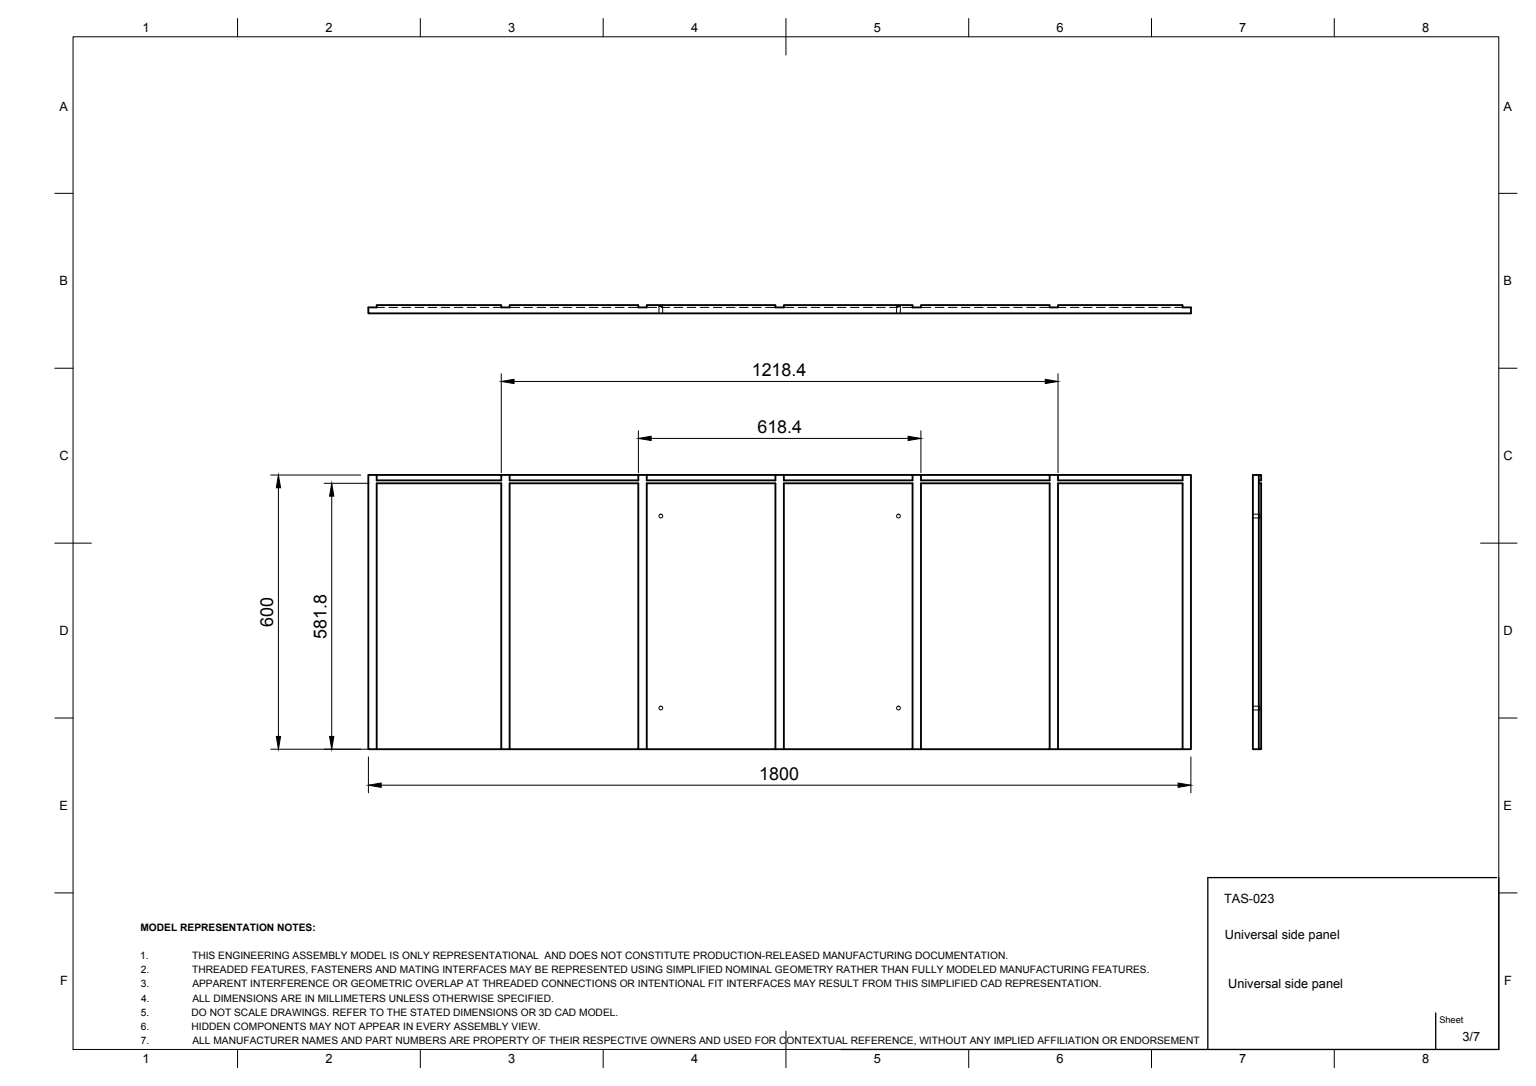
ISO-10303-21;
HEADER;
/* Generated by software containing ST-Developer
 * from STEP Tools, Inc. (www.steptools.com) 
 */

FILE_DESCRIPTION(
/* description */ (''),
/* implementation_level */ '2;1');

FILE_NAME(
/* name */ 'Universal side panel.step',
/* time_stamp */ '2026-11-15T17:51:54-08:00',
/* author */ (''),
/* organization */ (''),
/* preprocessor_version */ 'ST-DEVELOPER v20.2',
/* originating_system */ 'Autodesk Translation Framework v15.17.0.0',
/* authorisation */ '');

FILE_SCHEMA (('AUTOMOTIVE_DESIGN { 1 0 10303 214 3 1 1 }'));
ENDSEC;

DATA;
#10=MECHANICAL_DESIGN_GEOMETRIC_PRESENTATION_REPRESENTATION('',(#117),#2860);
#107=SHAPE_REPRESENTATION_RELATIONSHIP('SRR','None',#2902,#112);
#112=ADVANCED_BREP_SHAPE_REPRESENTATION('',(#122),#2855);
#117=STYLED_ITEM('',(#2936),#122);
#122=MANIFOLD_SOLID_BREP('Body1',#1714);
#127=FACE_BOUND('',#361,.T.);
#128=FACE_BOUND('',#362,.T.);
#129=FACE_BOUND('',#363,.T.);
#130=FACE_BOUND('',#364,.T.);
#131=PLANE('',#1780);
#132=PLANE('',#1784);
#133=PLANE('',#1788);
#134=PLANE('',#1792);
#135=PLANE('',#1793);
#136=PLANE('',#1794);
#137=PLANE('',#1795);
#138=PLANE('',#1796);
#139=PLANE('',#1797);
#140=PLANE('',#1798);
#141=PLANE('',#1799);
#142=PLANE('',#1800);
#143=PLANE('',#1801);
#144=PLANE('',#1802);
#145=PLANE('',#1803);
#146=PLANE('',#1804);
#147=PLANE('',#1805);
#148=PLANE('',#1806);
#149=PLANE('',#1807);
#150=PLANE('',#1808);
#151=PLANE('',#1809);
#152=PLANE('',#1810);
#153=PLANE('',#1811);
#154=PLANE('',#1812);
#155=PLANE('',#1813);
#156=PLANE('',#1814);
#157=PLANE('',#1815);
#158=PLANE('',#1816);
#159=PLANE('',#1817);
#160=PLANE('',#1818);
#161=PLANE('',#1819);
#162=PLANE('',#1820);
#163=PLANE('',#1821);
#164=PLANE('',#1822);
#165=PLANE('',#1823);
#166=PLANE('',#1824);
#167=PLANE('',#1825);
#168=PLANE('',#1826);
#169=PLANE('',#1827);
#170=PLANE('',#1828);
#171=PLANE('',#1829);
#172=PLANE('',#1830);
#173=PLANE('',#1831);
#174=PLANE('',#1832);
#175=PLANE('',#1833);
#176=PLANE('',#1834);
#177=PLANE('',#1835);
#178=PLANE('',#1836);
#179=PLANE('',#1837);
#180=PLANE('',#1838);
#181=PLANE('',#1839);
#182=PLANE('',#1840);
#183=PLANE('',#1841);
#184=PLANE('',#1842);
#185=PLANE('',#1843);
#186=PLANE('',#1844);
#187=PLANE('',#1845);
#188=PLANE('',#1846);
#213=FACE_OUTER_BOUND('',#300,.T.);
#214=FACE_OUTER_BOUND('',#301,.T.);
#215=FACE_OUTER_BOUND('',#302,.T.);
#216=FACE_OUTER_BOUND('',#303,.T.);
#217=FACE_OUTER_BOUND('',#304,.T.);
#218=FACE_OUTER_BOUND('',#305,.T.);
#219=FACE_OUTER_BOUND('',#306,.T.);
#220=FACE_OUTER_BOUND('',#307,.T.);
#221=FACE_OUTER_BOUND('',#308,.T.);
#222=FACE_OUTER_BOUND('',#309,.T.);
#223=FACE_OUTER_BOUND('',#310,.T.);
#224=FACE_OUTER_BOUND('',#311,.T.);
#225=FACE_OUTER_BOUND('',#312,.T.);
#226=FACE_OUTER_BOUND('',#313,.T.);
#227=FACE_OUTER_BOUND('',#314,.T.);
#228=FACE_OUTER_BOUND('',#315,.T.);
#229=FACE_OUTER_BOUND('',#316,.T.);
#230=FACE_OUTER_BOUND('',#317,.T.);
#231=FACE_OUTER_BOUND('',#318,.T.);
#232=FACE_OUTER_BOUND('',#319,.T.);
#233=FACE_OUTER_BOUND('',#320,.T.);
#234=FACE_OUTER_BOUND('',#321,.T.);
#235=FACE_OUTER_BOUND('',#322,.T.);
#236=FACE_OUTER_BOUND('',#323,.T.);
#237=FACE_OUTER_BOUND('',#324,.T.);
#238=FACE_OUTER_BOUND('',#325,.T.);
#239=FACE_OUTER_BOUND('',#326,.T.);
#240=FACE_OUTER_BOUND('',#327,.T.);
#241=FACE_OUTER_BOUND('',#328,.T.);
#242=FACE_OUTER_BOUND('',#329,.T.);
#243=FACE_OUTER_BOUND('',#330,.T.);
#244=FACE_OUTER_BOUND('',#331,.T.);
#245=FACE_OUTER_BOUND('',#332,.T.);
#246=FACE_OUTER_BOUND('',#333,.T.);
#247=FACE_OUTER_BOUND('',#334,.T.);
#248=FACE_OUTER_BOUND('',#335,.T.);
#249=FACE_OUTER_BOUND('',#336,.T.);
#250=FACE_OUTER_BOUND('',#337,.T.);
#251=FACE_OUTER_BOUND('',#338,.T.);
#252=FACE_OUTER_BOUND('',#339,.T.);
#253=FACE_OUTER_BOUND('',#340,.T.);
#254=FACE_OUTER_BOUND('',#341,.T.);
#255=FACE_OUTER_BOUND('',#342,.T.);
#256=FACE_OUTER_BOUND('',#343,.T.);
#257=FACE_OUTER_BOUND('',#344,.T.);
#258=FACE_OUTER_BOUND('',#345,.T.);
#259=FACE_OUTER_BOUND('',#346,.T.);
#260=FACE_OUTER_BOUND('',#347,.T.);
#261=FACE_OUTER_BOUND('',#348,.T.);
#262=FACE_OUTER_BOUND('',#349,.T.);
#263=FACE_OUTER_BOUND('',#350,.T.);
#264=FACE_OUTER_BOUND('',#351,.T.);
#265=FACE_OUTER_BOUND('',#352,.T.);
#266=FACE_OUTER_BOUND('',#353,.T.);
#267=FACE_OUTER_BOUND('',#354,.T.);
#268=FACE_OUTER_BOUND('',#355,.T.);
#269=FACE_OUTER_BOUND('',#356,.T.);
#270=FACE_OUTER_BOUND('',#357,.T.);
#271=FACE_OUTER_BOUND('',#358,.T.);
#272=FACE_OUTER_BOUND('',#359,.T.);
#273=FACE_OUTER_BOUND('',#360,.T.);
#274=FACE_OUTER_BOUND('',#365,.T.);
#300=EDGE_LOOP('',(#1184,#1185,#1186,#1187));
#301=EDGE_LOOP('',(#1188));
#302=EDGE_LOOP('',(#1189,#1190,#1191,#1192));
#303=EDGE_LOOP('',(#1193));
#304=EDGE_LOOP('',(#1194,#1195,#1196,#1197));
#305=EDGE_LOOP('',(#1198));
#306=EDGE_LOOP('',(#1199,#1200,#1201,#1202));
#307=EDGE_LOOP('',(#1203));
#308=EDGE_LOOP('',(#1204,#1205,#1206,#1207));
#309=EDGE_LOOP('',(#1208,#1209,#1210,#1211));
#310=EDGE_LOOP('',(#1212,#1213,#1214,#1215));
#311=EDGE_LOOP('',(#1216,#1217,#1218,#1219));
#312=EDGE_LOOP('',(#1220,#1221,#1222,#1223));
#313=EDGE_LOOP('',(#1224,#1225,#1226,#1227));
#314=EDGE_LOOP('',(#1228,#1229,#1230,#1231));
#315=EDGE_LOOP('',(#1232,#1233,#1234,#1235));
#316=EDGE_LOOP('',(#1236,#1237,#1238,#1239));
#317=EDGE_LOOP('',(#1240,#1241,#1242,#1243));
#318=EDGE_LOOP('',(#1244,#1245,#1246,#1247));
#319=EDGE_LOOP('',(#1248,#1249,#1250,#1251));
#320=EDGE_LOOP('',(#1252,#1253,#1254,#1255,#1256,#1257,#1258,#1259,#1260,
#1261,#1262,#1263,#1264,#1265,#1266,#1267,#1268,#1269,#1270,#1271,#1272,
#1273,#1274,#1275,#1276,#1277,#1278,#1279,#1280,#1281,#1282,#1283,#1284,
#1285,#1286,#1287,#1288,#1289,#1290,#1291,#1292,#1293,#1294,#1295,#1296,
#1297,#1298,#1299,#1300,#1301,#1302,#1303));
#321=EDGE_LOOP('',(#1304,#1305,#1306,#1307));
#322=EDGE_LOOP('',(#1308,#1309,#1310,#1311));
#323=EDGE_LOOP('',(#1312,#1313,#1314,#1315));
#324=EDGE_LOOP('',(#1316,#1317,#1318,#1319));
#325=EDGE_LOOP('',(#1320,#1321,#1322,#1323));
#326=EDGE_LOOP('',(#1324,#1325,#1326,#1327));
#327=EDGE_LOOP('',(#1328,#1329,#1330,#1331));
#328=EDGE_LOOP('',(#1332,#1333,#1334,#1335));
#329=EDGE_LOOP('',(#1336,#1337,#1338,#1339));
#330=EDGE_LOOP('',(#1340,#1341,#1342,#1343));
#331=EDGE_LOOP('',(#1344,#1345,#1346,#1347));
#332=EDGE_LOOP('',(#1348,#1349,#1350,#1351));
#333=EDGE_LOOP('',(#1352,#1353,#1354,#1355));
#334=EDGE_LOOP('',(#1356,#1357,#1358,#1359));
#335=EDGE_LOOP('',(#1360,#1361,#1362,#1363));
#336=EDGE_LOOP('',(#1364,#1365,#1366,#1367));
#337=EDGE_LOOP('',(#1368,#1369,#1370,#1371));
#338=EDGE_LOOP('',(#1372,#1373,#1374,#1375));
#339=EDGE_LOOP('',(#1376,#1377,#1378,#1379));
#340=EDGE_LOOP('',(#1380,#1381,#1382,#1383));
#341=EDGE_LOOP('',(#1384,#1385,#1386,#1387));
#342=EDGE_LOOP('',(#1388,#1389,#1390,#1391));
#343=EDGE_LOOP('',(#1392,#1393,#1394,#1395));
#344=EDGE_LOOP('',(#1396,#1397,#1398,#1399));
#345=EDGE_LOOP('',(#1400,#1401,#1402,#1403));
#346=EDGE_LOOP('',(#1404,#1405,#1406,#1407));
#347=EDGE_LOOP('',(#1408,#1409,#1410,#1411));
#348=EDGE_LOOP('',(#1412,#1413,#1414,#1415));
#349=EDGE_LOOP('',(#1416,#1417,#1418,#1419));
#350=EDGE_LOOP('',(#1420,#1421,#1422,#1423));
#351=EDGE_LOOP('',(#1424,#1425,#1426,#1427));
#352=EDGE_LOOP('',(#1428,#1429,#1430,#1431));
#353=EDGE_LOOP('',(#1432,#1433,#1434,#1435));
#354=EDGE_LOOP('',(#1436,#1437,#1438,#1439));
#355=EDGE_LOOP('',(#1440,#1441,#1442,#1443));
#356=EDGE_LOOP('',(#1444,#1445,#1446,#1447));
#357=EDGE_LOOP('',(#1448,#1449,#1450,#1451,#1452,#1453,#1454,#1455,#1456,
#1457,#1458,#1459,#1460,#1461,#1462,#1463,#1464,#1465,#1466,#1467,#1468,
#1469,#1470,#1471,#1472,#1473,#1474,#1475));
#358=EDGE_LOOP('',(#1476,#1477,#1478,#1479));
#359=EDGE_LOOP('',(#1480,#1481,#1482,#1483,#1484,#1485,#1486,#1487,#1488,
#1489,#1490,#1491,#1492,#1493,#1494,#1495,#1496,#1497,#1498,#1499,#1500,
#1501,#1502,#1503,#1504,#1505,#1506,#1507));
#360=EDGE_LOOP('',(#1508,#1509,#1510,#1511));
#361=EDGE_LOOP('',(#1512));
#362=EDGE_LOOP('',(#1513));
#363=EDGE_LOOP('',(#1514));
#364=EDGE_LOOP('',(#1515));
#365=EDGE_LOOP('',(#1516,#1517,#1518,#1519));
#391=LINE('',#2371,#600);
#392=LINE('',#2378,#601);
#393=LINE('',#2385,#602);
#394=LINE('',#2392,#603);
#395=LINE('',#2398,#604);
#396=LINE('',#2400,#605);
#397=LINE('',#2402,#606);
#398=LINE('',#2403,#607);
#399=LINE('',#2407,#608);
#400=LINE('',#2409,#609);
#401=LINE('',#2411,#610);
#402=LINE('',#2412,#611);
#403=LINE('',#2416,#612);
#404=LINE('',#2418,#613);
#405=LINE('',#2420,#614);
#406=LINE('',#2421,#615);
#407=LINE('',#2425,#616);
#408=LINE('',#2427,#617);
#409=LINE('',#2429,#618);
#410=LINE('',#2430,#619);
#411=LINE('',#2434,#620);
#412=LINE('',#2436,#621);
#413=LINE('',#2438,#622);
#414=LINE('',#2439,#623);
#415=LINE('',#2443,#624);
#416=LINE('',#2445,#625);
#417=LINE('',#2447,#626);
#418=LINE('',#2448,#627);
#419=LINE('',#2452,#628);
#420=LINE('',#2454,#629);
#421=LINE('',#2456,#630);
#422=LINE('',#2457,#631);
#423=LINE('',#2461,#632);
#424=LINE('',#2463,#633);
#425=LINE('',#2465,#634);
#426=LINE('',#2466,#635);
#427=LINE('',#2470,#636);
#428=LINE('',#2472,#637);
#429=LINE('',#2474,#638);
#430=LINE('',#2475,#639);
#431=LINE('',#2479,#640);
#432=LINE('',#2481,#641);
#433=LINE('',#2483,#642);
#434=LINE('',#2484,#643);
#435=LINE('',#2488,#644);
#436=LINE('',#2490,#645);
#437=LINE('',#2492,#646);
#438=LINE('',#2493,#647);
#439=LINE('',#2497,#648);
#440=LINE('',#2499,#649);
#441=LINE('',#2501,#650);
#442=LINE('',#2502,#651);
#443=LINE('',#2505,#652);
#444=LINE('',#2507,#653);
#445=LINE('',#2509,#654);
#446=LINE('',#2511,#655);
#447=LINE('',#2512,#656);
#448=LINE('',#2514,#657);
#449=LINE('',#2516,#658);
#450=LINE('',#2517,#659);
#451=LINE('',#2519,#660);
#452=LINE('',#2521,#661);
#453=LINE('',#2522,#662);
#454=LINE('',#2524,#663);
#455=LINE('',#2526,#664);
#456=LINE('',#2527,#665);
#457=LINE('',#2529,#666);
#458=LINE('',#2531,#667);
#459=LINE('',#2532,#668);
#460=LINE('',#2534,#669);
#461=LINE('',#2536,#670);
#462=LINE('',#2537,#671);
#463=LINE('',#2539,#672);
#464=LINE('',#2541,#673);
#465=LINE('',#2543,#674);
#466=LINE('',#2545,#675);
#467=LINE('',#2546,#676);
#468=LINE('',#2548,#677);
#469=LINE('',#2550,#678);
#470=LINE('',#2551,#679);
#471=LINE('',#2553,#680);
#472=LINE('',#2555,#681);
#473=LINE('',#2556,#682);
#474=LINE('',#2558,#683);
#475=LINE('',#2560,#684);
#476=LINE('',#2561,#685);
#477=LINE('',#2563,#686);
#478=LINE('',#2565,#687);
#479=LINE('',#2566,#688);
#480=LINE('',#2568,#689);
#481=LINE('',#2570,#690);
#482=LINE('',#2571,#691);
#483=LINE('',#2574,#692);
#484=LINE('',#2575,#693);
#485=LINE('',#2578,#694);
#486=LINE('',#2579,#695);
#487=LINE('',#2582,#696);
#488=LINE('',#2583,#697);
#489=LINE('',#2586,#698);
#490=LINE('',#2587,#699);
#491=LINE('',#2589,#700);
#492=LINE('',#2591,#701);
#493=LINE('',#2594,#702);
#494=LINE('',#2595,#703);
#495=LINE('',#2598,#704);
#496=LINE('',#2599,#705);
#497=LINE('',#2602,#706);
#498=LINE('',#2603,#707);
#499=LINE('',#2606,#708);
#500=LINE('',#2607,#709);
#501=LINE('',#2609,#710);
#502=LINE('',#2611,#711);
#503=LINE('',#2614,#712);
#504=LINE('',#2615,#713);
#505=LINE('',#2618,#714);
#506=LINE('',#2619,#715);
#507=LINE('',#2622,#716);
#508=LINE('',#2623,#717);
#509=LINE('',#2626,#718);
#510=LINE('',#2627,#719);
#511=LINE('',#2629,#720);
#512=LINE('',#2631,#721);
#513=LINE('',#2634,#722);
#514=LINE('',#2635,#723);
#515=LINE('',#2638,#724);
#516=LINE('',#2639,#725);
#517=LINE('',#2642,#726);
#518=LINE('',#2643,#727);
#519=LINE('',#2646,#728);
#520=LINE('',#2647,#729);
#521=LINE('',#2649,#730);
#522=LINE('',#2651,#731);
#523=LINE('',#2654,#732);
#524=LINE('',#2655,#733);
#525=LINE('',#2658,#734);
#526=LINE('',#2659,#735);
#527=LINE('',#2662,#736);
#528=LINE('',#2663,#737);
#529=LINE('',#2666,#738);
#530=LINE('',#2667,#739);
#531=LINE('',#2669,#740);
#532=LINE('',#2671,#741);
#533=LINE('',#2674,#742);
#534=LINE('',#2675,#743);
#535=LINE('',#2678,#744);
#536=LINE('',#2679,#745);
#537=LINE('',#2682,#746);
#538=LINE('',#2683,#747);
#539=LINE('',#2686,#748);
#540=LINE('',#2687,#749);
#541=LINE('',#2689,#750);
#542=LINE('',#2691,#751);
#543=LINE('',#2694,#752);
#544=LINE('',#2696,#753);
#545=LINE('',#2697,#754);
#546=LINE('',#2700,#755);
#547=LINE('',#2701,#756);
#548=LINE('',#2704,#757);
#549=LINE('',#2705,#758);
#550=LINE('',#2707,#759);
#600=VECTOR('',#1910,0.409999999999997);
#601=VECTOR('',#1919,0.409999999999997);
#602=VECTOR('',#1928,0.409999999999997);
#603=VECTOR('',#1937,0.409999999999997);
#604=VECTOR('',#1944,1.);
#605=VECTOR('',#1945,1.);
#606=VECTOR('',#1946,1.);
#607=VECTOR('',#1947,1.);
#608=VECTOR('',#1950,1.);
#609=VECTOR('',#1951,1.);
#610=VECTOR('',#1952,1.);
#611=VECTOR('',#1953,1.);
#612=VECTOR('',#1956,1.);
#613=VECTOR('',#1957,1.);
#614=VECTOR('',#1958,1.);
#615=VECTOR('',#1959,1.);
#616=VECTOR('',#1962,1.);
#617=VECTOR('',#1963,1.);
#618=VECTOR('',#1964,1.);
#619=VECTOR('',#1965,1.);
#620=VECTOR('',#1968,1.);
#621=VECTOR('',#1969,1.);
#622=VECTOR('',#1970,1.);
#623=VECTOR('',#1971,1.);
#624=VECTOR('',#1974,1.);
#625=VECTOR('',#1975,1.);
#626=VECTOR('',#1976,1.);
#627=VECTOR('',#1977,1.);
#628=VECTOR('',#1980,1.);
#629=VECTOR('',#1981,1.);
#630=VECTOR('',#1982,1.);
#631=VECTOR('',#1983,1.);
#632=VECTOR('',#1986,1.);
#633=VECTOR('',#1987,1.);
#634=VECTOR('',#1988,1.);
#635=VECTOR('',#1989,1.);
#636=VECTOR('',#1992,1.);
#637=VECTOR('',#1993,1.);
#638=VECTOR('',#1994,1.);
#639=VECTOR('',#1995,1.);
#640=VECTOR('',#1998,1.);
#641=VECTOR('',#1999,1.);
#642=VECTOR('',#2000,1.);
#643=VECTOR('',#2001,1.);
#644=VECTOR('',#2004,1.);
#645=VECTOR('',#2005,1.);
#646=VECTOR('',#2006,1.);
#647=VECTOR('',#2007,1.);
#648=VECTOR('',#2010,1.);
#649=VECTOR('',#2011,1.);
#650=VECTOR('',#2012,1.);
#651=VECTOR('',#2013,1.);
#652=VECTOR('',#2016,1.);
#653=VECTOR('',#2017,1.);
#654=VECTOR('',#2018,1.);
#655=VECTOR('',#2019,1.);
#656=VECTOR('',#2020,1.);
#657=VECTOR('',#2021,1.);
#658=VECTOR('',#2022,1.);
#659=VECTOR('',#2023,1.);
#660=VECTOR('',#2024,1.);
#661=VECTOR('',#2025,1.);
#662=VECTOR('',#2026,1.);
#663=VECTOR('',#2027,1.);
#664=VECTOR('',#2028,1.);
#665=VECTOR('',#2029,1.);
#666=VECTOR('',#2030,1.);
#667=VECTOR('',#2031,1.);
#668=VECTOR('',#2032,1.);
#669=VECTOR('',#2033,1.);
#670=VECTOR('',#2034,1.);
#671=VECTOR('',#2035,1.);
#672=VECTOR('',#2036,1.);
#673=VECTOR('',#2037,1.);
#674=VECTOR('',#2038,1.);
#675=VECTOR('',#2039,1.);
#676=VECTOR('',#2040,1.);
#677=VECTOR('',#2041,1.);
#678=VECTOR('',#2042,1.);
#679=VECTOR('',#2043,1.);
#680=VECTOR('',#2044,1.);
#681=VECTOR('',#2045,1.);
#682=VECTOR('',#2046,1.);
#683=VECTOR('',#2047,1.);
#684=VECTOR('',#2048,1.);
#685=VECTOR('',#2049,1.);
#686=VECTOR('',#2050,1.);
#687=VECTOR('',#2051,1.);
#688=VECTOR('',#2052,1.);
#689=VECTOR('',#2053,1.);
#690=VECTOR('',#2054,1.);
#691=VECTOR('',#2055,1.);
#692=VECTOR('',#2058,1.);
#693=VECTOR('',#2059,1.);
#694=VECTOR('',#2062,1.);
#695=VECTOR('',#2063,1.);
#696=VECTOR('',#2066,1.);
#697=VECTOR('',#2067,1.);
#698=VECTOR('',#2070,1.);
#699=VECTOR('',#2071,1.);
#700=VECTOR('',#2074,1.);
#701=VECTOR('',#2077,1.);
#702=VECTOR('',#2080,1.);
#703=VECTOR('',#2081,1.);
#704=VECTOR('',#2084,1.);
#705=VECTOR('',#2085,1.);
#706=VECTOR('',#2088,1.);
#707=VECTOR('',#2089,1.);
#708=VECTOR('',#2092,1.);
#709=VECTOR('',#2093,1.);
#710=VECTOR('',#2096,1.);
#711=VECTOR('',#2099,1.);
#712=VECTOR('',#2102,1.);
#713=VECTOR('',#2103,1.);
#714=VECTOR('',#2106,1.);
#715=VECTOR('',#2107,1.);
#716=VECTOR('',#2110,1.);
#717=VECTOR('',#2111,1.);
#718=VECTOR('',#2114,1.);
#719=VECTOR('',#2115,1.);
#720=VECTOR('',#2118,1.);
#721=VECTOR('',#2121,1.);
#722=VECTOR('',#2124,1.);
#723=VECTOR('',#2125,1.);
#724=VECTOR('',#2128,1.);
#725=VECTOR('',#2129,1.);
#726=VECTOR('',#2132,1.);
#727=VECTOR('',#2133,1.);
#728=VECTOR('',#2136,1.);
#729=VECTOR('',#2137,1.);
#730=VECTOR('',#2140,1.);
#731=VECTOR('',#2143,1.);
#732=VECTOR('',#2146,1.);
#733=VECTOR('',#2147,1.);
#734=VECTOR('',#2150,1.);
#735=VECTOR('',#2151,1.);
#736=VECTOR('',#2154,1.);
#737=VECTOR('',#2155,1.);
#738=VECTOR('',#2158,1.);
#739=VECTOR('',#2159,1.);
#740=VECTOR('',#2162,1.);
#741=VECTOR('',#2165,1.);
#742=VECTOR('',#2168,1.);
#743=VECTOR('',#2169,1.);
#744=VECTOR('',#2172,1.);
#745=VECTOR('',#2173,1.);
#746=VECTOR('',#2176,1.);
#747=VECTOR('',#2177,1.);
#748=VECTOR('',#2180,1.);
#749=VECTOR('',#2181,1.);
#750=VECTOR('',#2184,1.);
#751=VECTOR('',#2187,1.);
#752=VECTOR('',#2190,1.);
#753=VECTOR('',#2191,1.);
#754=VECTOR('',#2192,1.);
#755=VECTOR('',#2195,1.);
#756=VECTOR('',#2196,1.);
#757=VECTOR('',#2199,1.);
#758=VECTOR('',#2200,1.);
#759=VECTOR('',#2203,1.);
#809=CIRCLE('',#1778,0.409999999999997);
#810=CIRCLE('',#1779,0.409999999999997);
#811=CIRCLE('',#1782,0.409999999999997);
#812=CIRCLE('',#1783,0.409999999999997);
#813=CIRCLE('',#1786,0.409999999999997);
#814=CIRCLE('',#1787,0.409999999999997);
#815=CIRCLE('',#1790,0.409999999999997);
#816=CIRCLE('',#1791,0.409999999999997);
#819=VERTEX_POINT('',#2368);
#820=VERTEX_POINT('',#2370);
#821=VERTEX_POINT('',#2375);
#822=VERTEX_POINT('',#2377);
#823=VERTEX_POINT('',#2382);
#824=VERTEX_POINT('',#2384);
#825=VERTEX_POINT('',#2389);
#826=VERTEX_POINT('',#2391);
#827=VERTEX_POINT('',#2396);
#828=VERTEX_POINT('',#2397);
#829=VERTEX_POINT('',#2399);
#830=VERTEX_POINT('',#2401);
#831=VERTEX_POINT('',#2405);
#832=VERTEX_POINT('',#2406);
#833=VERTEX_POINT('',#2408);
#834=VERTEX_POINT('',#2410);
#835=VERTEX_POINT('',#2414);
#836=VERTEX_POINT('',#2415);
#837=VERTEX_POINT('',#2417);
#838=VERTEX_POINT('',#2419);
#839=VERTEX_POINT('',#2423);
#840=VERTEX_POINT('',#2424);
#841=VERTEX_POINT('',#2426);
#842=VERTEX_POINT('',#2428);
#843=VERTEX_POINT('',#2432);
#844=VERTEX_POINT('',#2433);
#845=VERTEX_POINT('',#2435);
#846=VERTEX_POINT('',#2437);
#847=VERTEX_POINT('',#2441);
#848=VERTEX_POINT('',#2442);
#849=VERTEX_POINT('',#2444);
#850=VERTEX_POINT('',#2446);
#851=VERTEX_POINT('',#2450);
#852=VERTEX_POINT('',#2451);
#853=VERTEX_POINT('',#2453);
#854=VERTEX_POINT('',#2455);
#855=VERTEX_POINT('',#2459);
#856=VERTEX_POINT('',#2460);
#857=VERTEX_POINT('',#2462);
#858=VERTEX_POINT('',#2464);
#859=VERTEX_POINT('',#2468);
#860=VERTEX_POINT('',#2469);
#861=VERTEX_POINT('',#2471);
#862=VERTEX_POINT('',#2473);
#863=VERTEX_POINT('',#2477);
#864=VERTEX_POINT('',#2478);
#865=VERTEX_POINT('',#2480);
#866=VERTEX_POINT('',#2482);
#867=VERTEX_POINT('',#2486);
#868=VERTEX_POINT('',#2487);
#869=VERTEX_POINT('',#2489);
#870=VERTEX_POINT('',#2491);
#871=VERTEX_POINT('',#2495);
#872=VERTEX_POINT('',#2496);
#873=VERTEX_POINT('',#2498);
#874=VERTEX_POINT('',#2500);
#875=VERTEX_POINT('',#2504);
#876=VERTEX_POINT('',#2506);
#877=VERTEX_POINT('',#2508);
#878=VERTEX_POINT('',#2510);
#879=VERTEX_POINT('',#2513);
#880=VERTEX_POINT('',#2515);
#881=VERTEX_POINT('',#2518);
#882=VERTEX_POINT('',#2520);
#883=VERTEX_POINT('',#2523);
#884=VERTEX_POINT('',#2525);
#885=VERTEX_POINT('',#2528);
#886=VERTEX_POINT('',#2530);
#887=VERTEX_POINT('',#2533);
#888=VERTEX_POINT('',#2535);
#889=VERTEX_POINT('',#2538);
#890=VERTEX_POINT('',#2540);
#891=VERTEX_POINT('',#2542);
#892=VERTEX_POINT('',#2544);
#893=VERTEX_POINT('',#2547);
#894=VERTEX_POINT('',#2549);
#895=VERTEX_POINT('',#2552);
#896=VERTEX_POINT('',#2554);
#897=VERTEX_POINT('',#2557);
#898=VERTEX_POINT('',#2559);
#899=VERTEX_POINT('',#2562);
#900=VERTEX_POINT('',#2564);
#901=VERTEX_POINT('',#2567);
#902=VERTEX_POINT('',#2569);
#903=VERTEX_POINT('',#2573);
#904=VERTEX_POINT('',#2577);
#905=VERTEX_POINT('',#2581);
#906=VERTEX_POINT('',#2585);
#907=VERTEX_POINT('',#2593);
#908=VERTEX_POINT('',#2597);
#909=VERTEX_POINT('',#2601);
#910=VERTEX_POINT('',#2605);
#911=VERTEX_POINT('',#2613);
#912=VERTEX_POINT('',#2617);
#913=VERTEX_POINT('',#2621);
#914=VERTEX_POINT('',#2625);
#915=VERTEX_POINT('',#2633);
#916=VERTEX_POINT('',#2637);
#917=VERTEX_POINT('',#2641);
#918=VERTEX_POINT('',#2645);
#919=VERTEX_POINT('',#2653);
#920=VERTEX_POINT('',#2657);
#921=VERTEX_POINT('',#2661);
#922=VERTEX_POINT('',#2665);
#923=VERTEX_POINT('',#2673);
#924=VERTEX_POINT('',#2677);
#925=VERTEX_POINT('',#2681);
#926=VERTEX_POINT('',#2685);
#927=VERTEX_POINT('',#2693);
#928=VERTEX_POINT('',#2695);
#929=VERTEX_POINT('',#2699);
#930=VERTEX_POINT('',#2703);
#965=EDGE_CURVE('',#819,#819,#809,.T.);
#966=EDGE_CURVE('',#819,#820,#391,.T.);
#967=EDGE_CURVE('',#820,#820,#810,.T.);
#968=EDGE_CURVE('',#821,#821,#811,.T.);
#969=EDGE_CURVE('',#821,#822,#392,.T.);
#970=EDGE_CURVE('',#822,#822,#812,.T.);
#971=EDGE_CURVE('',#823,#823,#813,.T.);
#972=EDGE_CURVE('',#823,#824,#393,.T.);
#973=EDGE_CURVE('',#824,#824,#814,.T.);
#974=EDGE_CURVE('',#825,#825,#815,.T.);
#975=EDGE_CURVE('',#825,#826,#394,.T.);
#976=EDGE_CURVE('',#826,#826,#816,.T.);
#977=EDGE_CURVE('',#827,#828,#395,.T.);
#978=EDGE_CURVE('',#829,#827,#396,.T.);
#979=EDGE_CURVE('',#830,#829,#397,.T.);
#980=EDGE_CURVE('',#828,#830,#398,.T.);
#981=EDGE_CURVE('',#831,#832,#399,.T.);
#982=EDGE_CURVE('',#833,#831,#400,.T.);
#983=EDGE_CURVE('',#834,#833,#401,.T.);
#984=EDGE_CURVE('',#832,#834,#402,.T.);
#985=EDGE_CURVE('',#835,#836,#403,.T.);
#986=EDGE_CURVE('',#837,#835,#404,.T.);
#987=EDGE_CURVE('',#838,#837,#405,.T.);
#988=EDGE_CURVE('',#836,#838,#406,.T.);
#989=EDGE_CURVE('',#839,#840,#407,.T.);
#990=EDGE_CURVE('',#841,#839,#408,.T.);
#991=EDGE_CURVE('',#842,#841,#409,.T.);
#992=EDGE_CURVE('',#840,#842,#410,.T.);
#993=EDGE_CURVE('',#843,#844,#411,.T.);
#994=EDGE_CURVE('',#845,#843,#412,.T.);
#995=EDGE_CURVE('',#846,#845,#413,.T.);
#996=EDGE_CURVE('',#844,#846,#414,.T.);
#997=EDGE_CURVE('',#847,#848,#415,.T.);
#998=EDGE_CURVE('',#849,#847,#416,.T.);
#999=EDGE_CURVE('',#850,#849,#417,.T.);
#1000=EDGE_CURVE('',#848,#850,#418,.T.);
#1001=EDGE_CURVE('',#851,#852,#419,.T.);
#1002=EDGE_CURVE('',#853,#851,#420,.T.);
#1003=EDGE_CURVE('',#854,#853,#421,.T.);
#1004=EDGE_CURVE('',#854,#852,#422,.T.);
#1005=EDGE_CURVE('',#855,#856,#423,.T.);
#1006=EDGE_CURVE('',#857,#855,#424,.T.);
#1007=EDGE_CURVE('',#858,#857,#425,.T.);
#1008=EDGE_CURVE('',#858,#856,#426,.T.);
#1009=EDGE_CURVE('',#859,#860,#427,.T.);
#1010=EDGE_CURVE('',#861,#859,#428,.T.);
#1011=EDGE_CURVE('',#862,#861,#429,.T.);
#1012=EDGE_CURVE('',#862,#860,#430,.T.);
#1013=EDGE_CURVE('',#863,#864,#431,.T.);
#1014=EDGE_CURVE('',#865,#863,#432,.T.);
#1015=EDGE_CURVE('',#866,#865,#433,.T.);
#1016=EDGE_CURVE('',#866,#864,#434,.T.);
#1017=EDGE_CURVE('',#867,#868,#435,.T.);
#1018=EDGE_CURVE('',#869,#867,#436,.T.);
#1019=EDGE_CURVE('',#870,#869,#437,.T.);
#1020=EDGE_CURVE('',#870,#868,#438,.T.);
#1021=EDGE_CURVE('',#871,#872,#439,.T.);
#1022=EDGE_CURVE('',#873,#871,#440,.T.);
#1023=EDGE_CURVE('',#874,#873,#441,.T.);
#1024=EDGE_CURVE('',#874,#872,#442,.T.);
#1025=EDGE_CURVE('',#875,#847,#443,.T.);
#1026=EDGE_CURVE('',#876,#875,#444,.T.);
#1027=EDGE_CURVE('',#877,#876,#445,.T.);
#1028=EDGE_CURVE('',#878,#877,#446,.T.);
#1029=EDGE_CURVE('',#872,#878,#447,.T.);
#1030=EDGE_CURVE('',#874,#879,#448,.T.);
#1031=EDGE_CURVE('',#880,#879,#449,.T.);
#1032=EDGE_CURVE('',#868,#880,#450,.T.);
#1033=EDGE_CURVE('',#870,#881,#451,.T.);
#1034=EDGE_CURVE('',#882,#881,#452,.T.);
#1035=EDGE_CURVE('',#864,#882,#453,.T.);
#1036=EDGE_CURVE('',#866,#883,#454,.T.);
#1037=EDGE_CURVE('',#884,#883,#455,.T.);
#1038=EDGE_CURVE('',#860,#884,#456,.T.);
#1039=EDGE_CURVE('',#862,#885,#457,.T.);
#1040=EDGE_CURVE('',#886,#885,#458,.T.);
#1041=EDGE_CURVE('',#856,#886,#459,.T.);
#1042=EDGE_CURVE('',#858,#887,#460,.T.);
#1043=EDGE_CURVE('',#888,#887,#461,.T.);
#1044=EDGE_CURVE('',#852,#888,#462,.T.);
#1045=EDGE_CURVE('',#854,#889,#463,.T.);
#1046=EDGE_CURVE('',#890,#889,#464,.T.);
#1047=EDGE_CURVE('',#891,#890,#465,.T.);
#1048=EDGE_CURVE('',#892,#891,#466,.T.);
#1049=EDGE_CURVE('',#892,#845,#467,.T.);
#1050=EDGE_CURVE('',#893,#843,#468,.T.);
#1051=EDGE_CURVE('',#894,#893,#469,.T.);
#1052=EDGE_CURVE('',#894,#841,#470,.T.);
#1053=EDGE_CURVE('',#895,#839,#471,.T.);
#1054=EDGE_CURVE('',#896,#895,#472,.T.);
#1055=EDGE_CURVE('',#896,#837,#473,.T.);
#1056=EDGE_CURVE('',#897,#835,#474,.T.);
#1057=EDGE_CURVE('',#898,#897,#475,.T.);
#1058=EDGE_CURVE('',#898,#833,#476,.T.);
#1059=EDGE_CURVE('',#899,#831,#477,.T.);
#1060=EDGE_CURVE('',#900,#899,#478,.T.);
#1061=EDGE_CURVE('',#900,#829,#479,.T.);
#1062=EDGE_CURVE('',#901,#827,#480,.T.);
#1063=EDGE_CURVE('',#902,#901,#481,.T.);
#1064=EDGE_CURVE('',#902,#849,#482,.T.);
#1065=EDGE_CURVE('',#903,#878,#483,.T.);
#1066=EDGE_CURVE('',#871,#903,#484,.T.);
#1067=EDGE_CURVE('',#904,#848,#485,.T.);
#1068=EDGE_CURVE('',#875,#904,#486,.T.);
#1069=EDGE_CURVE('',#905,#903,#487,.T.);
#1070=EDGE_CURVE('',#905,#873,#488,.T.);
#1071=EDGE_CURVE('',#850,#906,#489,.T.);
#1072=EDGE_CURVE('',#906,#904,#490,.T.);
#1073=EDGE_CURVE('',#879,#905,#491,.T.);
#1074=EDGE_CURVE('',#906,#902,#492,.T.);
#1075=EDGE_CURVE('',#907,#880,#493,.T.);
#1076=EDGE_CURVE('',#867,#907,#494,.T.);
#1077=EDGE_CURVE('',#908,#828,#495,.T.);
#1078=EDGE_CURVE('',#901,#908,#496,.T.);
#1079=EDGE_CURVE('',#909,#907,#497,.T.);
#1080=EDGE_CURVE('',#909,#869,#498,.T.);
#1081=EDGE_CURVE('',#830,#910,#499,.T.);
#1082=EDGE_CURVE('',#910,#908,#500,.T.);
#1083=EDGE_CURVE('',#881,#909,#501,.T.);
#1084=EDGE_CURVE('',#910,#900,#502,.T.);
#1085=EDGE_CURVE('',#911,#882,#503,.T.);
#1086=EDGE_CURVE('',#863,#911,#504,.T.);
#1087=EDGE_CURVE('',#912,#832,#505,.T.);
#1088=EDGE_CURVE('',#899,#912,#506,.T.);
#1089=EDGE_CURVE('',#913,#911,#507,.T.);
#1090=EDGE_CURVE('',#913,#865,#508,.T.);
#1091=EDGE_CURVE('',#834,#914,#509,.T.);
#1092=EDGE_CURVE('',#914,#912,#510,.T.);
#1093=EDGE_CURVE('',#883,#913,#511,.T.);
#1094=EDGE_CURVE('',#914,#898,#512,.T.);
#1095=EDGE_CURVE('',#915,#884,#513,.T.);
#1096=EDGE_CURVE('',#859,#915,#514,.T.);
#1097=EDGE_CURVE('',#916,#836,#515,.T.);
#1098=EDGE_CURVE('',#897,#916,#516,.T.);
#1099=EDGE_CURVE('',#917,#915,#517,.T.);
#1100=EDGE_CURVE('',#917,#861,#518,.T.);
#1101=EDGE_CURVE('',#838,#918,#519,.T.);
#1102=EDGE_CURVE('',#918,#916,#520,.T.);
#1103=EDGE_CURVE('',#885,#917,#521,.T.);
#1104=EDGE_CURVE('',#918,#896,#522,.T.);
#1105=EDGE_CURVE('',#919,#886,#523,.T.);
#1106=EDGE_CURVE('',#855,#919,#524,.T.);
#1107=EDGE_CURVE('',#920,#840,#525,.T.);
#1108=EDGE_CURVE('',#895,#920,#526,.T.);
#1109=EDGE_CURVE('',#921,#919,#527,.T.);
#1110=EDGE_CURVE('',#921,#857,#528,.T.);
#1111=EDGE_CURVE('',#842,#922,#529,.T.);
#1112=EDGE_CURVE('',#922,#920,#530,.T.);
#1113=EDGE_CURVE('',#887,#921,#531,.T.);
#1114=EDGE_CURVE('',#922,#894,#532,.T.);
#1115=EDGE_CURVE('',#923,#888,#533,.T.);
#1116=EDGE_CURVE('',#851,#923,#534,.T.);
#1117=EDGE_CURVE('',#924,#844,#535,.T.);
#1118=EDGE_CURVE('',#893,#924,#536,.T.);
#1119=EDGE_CURVE('',#925,#923,#537,.T.);
#1120=EDGE_CURVE('',#925,#853,#538,.T.);
#1121=EDGE_CURVE('',#846,#926,#539,.T.);
#1122=EDGE_CURVE('',#926,#924,#540,.T.);
#1123=EDGE_CURVE('',#889,#925,#541,.T.);
#1124=EDGE_CURVE('',#926,#892,#542,.T.);
#1125=EDGE_CURVE('',#891,#927,#543,.T.);
#1126=EDGE_CURVE('',#927,#928,#544,.T.);
#1127=EDGE_CURVE('',#876,#928,#545,.T.);
#1128=EDGE_CURVE('',#929,#890,#546,.T.);
#1129=EDGE_CURVE('',#927,#929,#547,.T.);
#1130=EDGE_CURVE('',#930,#877,#548,.T.);
#1131=EDGE_CURVE('',#929,#930,#549,.T.);
#1132=EDGE_CURVE('',#928,#930,#550,.T.);
#1184=ORIENTED_EDGE('',*,*,#965,.F.);
#1185=ORIENTED_EDGE('',*,*,#966,.T.);
#1186=ORIENTED_EDGE('',*,*,#967,.T.);
#1187=ORIENTED_EDGE('',*,*,#966,.F.);
#1188=ORIENTED_EDGE('',*,*,#967,.F.);
#1189=ORIENTED_EDGE('',*,*,#968,.F.);
#1190=ORIENTED_EDGE('',*,*,#969,.T.);
#1191=ORIENTED_EDGE('',*,*,#970,.T.);
#1192=ORIENTED_EDGE('',*,*,#969,.F.);
#1193=ORIENTED_EDGE('',*,*,#970,.F.);
#1194=ORIENTED_EDGE('',*,*,#971,.F.);
#1195=ORIENTED_EDGE('',*,*,#972,.T.);
#1196=ORIENTED_EDGE('',*,*,#973,.T.);
#1197=ORIENTED_EDGE('',*,*,#972,.F.);
#1198=ORIENTED_EDGE('',*,*,#973,.F.);
#1199=ORIENTED_EDGE('',*,*,#974,.F.);
#1200=ORIENTED_EDGE('',*,*,#975,.T.);
#1201=ORIENTED_EDGE('',*,*,#976,.T.);
#1202=ORIENTED_EDGE('',*,*,#975,.F.);
#1203=ORIENTED_EDGE('',*,*,#976,.F.);
#1204=ORIENTED_EDGE('',*,*,#977,.F.);
#1205=ORIENTED_EDGE('',*,*,#978,.F.);
#1206=ORIENTED_EDGE('',*,*,#979,.F.);
#1207=ORIENTED_EDGE('',*,*,#980,.F.);
#1208=ORIENTED_EDGE('',*,*,#981,.F.);
#1209=ORIENTED_EDGE('',*,*,#982,.F.);
#1210=ORIENTED_EDGE('',*,*,#983,.F.);
#1211=ORIENTED_EDGE('',*,*,#984,.F.);
#1212=ORIENTED_EDGE('',*,*,#985,.F.);
#1213=ORIENTED_EDGE('',*,*,#986,.F.);
#1214=ORIENTED_EDGE('',*,*,#987,.F.);
#1215=ORIENTED_EDGE('',*,*,#988,.F.);
#1216=ORIENTED_EDGE('',*,*,#989,.F.);
#1217=ORIENTED_EDGE('',*,*,#990,.F.);
#1218=ORIENTED_EDGE('',*,*,#991,.F.);
#1219=ORIENTED_EDGE('',*,*,#992,.F.);
#1220=ORIENTED_EDGE('',*,*,#993,.F.);
#1221=ORIENTED_EDGE('',*,*,#994,.F.);
#1222=ORIENTED_EDGE('',*,*,#995,.F.);
#1223=ORIENTED_EDGE('',*,*,#996,.F.);
#1224=ORIENTED_EDGE('',*,*,#997,.F.);
#1225=ORIENTED_EDGE('',*,*,#998,.F.);
#1226=ORIENTED_EDGE('',*,*,#999,.F.);
#1227=ORIENTED_EDGE('',*,*,#1000,.F.);
#1228=ORIENTED_EDGE('',*,*,#1001,.F.);
#1229=ORIENTED_EDGE('',*,*,#1002,.F.);
#1230=ORIENTED_EDGE('',*,*,#1003,.F.);
#1231=ORIENTED_EDGE('',*,*,#1004,.T.);
#1232=ORIENTED_EDGE('',*,*,#1005,.F.);
#1233=ORIENTED_EDGE('',*,*,#1006,.F.);
#1234=ORIENTED_EDGE('',*,*,#1007,.F.);
#1235=ORIENTED_EDGE('',*,*,#1008,.T.);
#1236=ORIENTED_EDGE('',*,*,#1009,.F.);
#1237=ORIENTED_EDGE('',*,*,#1010,.F.);
#1238=ORIENTED_EDGE('',*,*,#1011,.F.);
#1239=ORIENTED_EDGE('',*,*,#1012,.T.);
#1240=ORIENTED_EDGE('',*,*,#1013,.F.);
#1241=ORIENTED_EDGE('',*,*,#1014,.F.);
#1242=ORIENTED_EDGE('',*,*,#1015,.F.);
#1243=ORIENTED_EDGE('',*,*,#1016,.T.);
#1244=ORIENTED_EDGE('',*,*,#1017,.F.);
#1245=ORIENTED_EDGE('',*,*,#1018,.F.);
#1246=ORIENTED_EDGE('',*,*,#1019,.F.);
#1247=ORIENTED_EDGE('',*,*,#1020,.T.);
#1248=ORIENTED_EDGE('',*,*,#1021,.F.);
#1249=ORIENTED_EDGE('',*,*,#1022,.F.);
#1250=ORIENTED_EDGE('',*,*,#1023,.F.);
#1251=ORIENTED_EDGE('',*,*,#1024,.T.);
#1252=ORIENTED_EDGE('',*,*,#1025,.F.);
#1253=ORIENTED_EDGE('',*,*,#1026,.F.);
#1254=ORIENTED_EDGE('',*,*,#1027,.F.);
#1255=ORIENTED_EDGE('',*,*,#1028,.F.);
#1256=ORIENTED_EDGE('',*,*,#1029,.F.);
#1257=ORIENTED_EDGE('',*,*,#1024,.F.);
#1258=ORIENTED_EDGE('',*,*,#1030,.T.);
#1259=ORIENTED_EDGE('',*,*,#1031,.F.);
#1260=ORIENTED_EDGE('',*,*,#1032,.F.);
#1261=ORIENTED_EDGE('',*,*,#1020,.F.);
#1262=ORIENTED_EDGE('',*,*,#1033,.T.);
#1263=ORIENTED_EDGE('',*,*,#1034,.F.);
#1264=ORIENTED_EDGE('',*,*,#1035,.F.);
#1265=ORIENTED_EDGE('',*,*,#1016,.F.);
#1266=ORIENTED_EDGE('',*,*,#1036,.T.);
#1267=ORIENTED_EDGE('',*,*,#1037,.F.);
#1268=ORIENTED_EDGE('',*,*,#1038,.F.);
#1269=ORIENTED_EDGE('',*,*,#1012,.F.);
#1270=ORIENTED_EDGE('',*,*,#1039,.T.);
#1271=ORIENTED_EDGE('',*,*,#1040,.F.);
#1272=ORIENTED_EDGE('',*,*,#1041,.F.);
#1273=ORIENTED_EDGE('',*,*,#1008,.F.);
#1274=ORIENTED_EDGE('',*,*,#1042,.T.);
#1275=ORIENTED_EDGE('',*,*,#1043,.F.);
#1276=ORIENTED_EDGE('',*,*,#1044,.F.);
#1277=ORIENTED_EDGE('',*,*,#1004,.F.);
#1278=ORIENTED_EDGE('',*,*,#1045,.T.);
#1279=ORIENTED_EDGE('',*,*,#1046,.F.);
#1280=ORIENTED_EDGE('',*,*,#1047,.F.);
#1281=ORIENTED_EDGE('',*,*,#1048,.F.);
#1282=ORIENTED_EDGE('',*,*,#1049,.T.);
#1283=ORIENTED_EDGE('',*,*,#994,.T.);
#1284=ORIENTED_EDGE('',*,*,#1050,.F.);
#1285=ORIENTED_EDGE('',*,*,#1051,.F.);
#1286=ORIENTED_EDGE('',*,*,#1052,.T.);
#1287=ORIENTED_EDGE('',*,*,#990,.T.);
#1288=ORIENTED_EDGE('',*,*,#1053,.F.);
#1289=ORIENTED_EDGE('',*,*,#1054,.F.);
#1290=ORIENTED_EDGE('',*,*,#1055,.T.);
#1291=ORIENTED_EDGE('',*,*,#986,.T.);
#1292=ORIENTED_EDGE('',*,*,#1056,.F.);
#1293=ORIENTED_EDGE('',*,*,#1057,.F.);
#1294=ORIENTED_EDGE('',*,*,#1058,.T.);
#1295=ORIENTED_EDGE('',*,*,#982,.T.);
#1296=ORIENTED_EDGE('',*,*,#1059,.F.);
#1297=ORIENTED_EDGE('',*,*,#1060,.F.);
#1298=ORIENTED_EDGE('',*,*,#1061,.T.);
#1299=ORIENTED_EDGE('',*,*,#978,.T.);
#1300=ORIENTED_EDGE('',*,*,#1062,.F.);
#1301=ORIENTED_EDGE('',*,*,#1063,.F.);
#1302=ORIENTED_EDGE('',*,*,#1064,.T.);
#1303=ORIENTED_EDGE('',*,*,#998,.T.);
#1304=ORIENTED_EDGE('',*,*,#1021,.T.);
#1305=ORIENTED_EDGE('',*,*,#1029,.T.);
#1306=ORIENTED_EDGE('',*,*,#1065,.F.);
#1307=ORIENTED_EDGE('',*,*,#1066,.F.);
#1308=ORIENTED_EDGE('',*,*,#997,.T.);
#1309=ORIENTED_EDGE('',*,*,#1067,.F.);
#1310=ORIENTED_EDGE('',*,*,#1068,.F.);
#1311=ORIENTED_EDGE('',*,*,#1025,.T.);
#1312=ORIENTED_EDGE('',*,*,#1022,.T.);
#1313=ORIENTED_EDGE('',*,*,#1066,.T.);
#1314=ORIENTED_EDGE('',*,*,#1069,.F.);
#1315=ORIENTED_EDGE('',*,*,#1070,.T.);
#1316=ORIENTED_EDGE('',*,*,#1000,.T.);
#1317=ORIENTED_EDGE('',*,*,#1071,.T.);
#1318=ORIENTED_EDGE('',*,*,#1072,.T.);
#1319=ORIENTED_EDGE('',*,*,#1067,.T.);
#1320=ORIENTED_EDGE('',*,*,#1023,.T.);
#1321=ORIENTED_EDGE('',*,*,#1070,.F.);
#1322=ORIENTED_EDGE('',*,*,#1073,.F.);
#1323=ORIENTED_EDGE('',*,*,#1030,.F.);
#1324=ORIENTED_EDGE('',*,*,#999,.T.);
#1325=ORIENTED_EDGE('',*,*,#1064,.F.);
#1326=ORIENTED_EDGE('',*,*,#1074,.F.);
#1327=ORIENTED_EDGE('',*,*,#1071,.F.);
#1328=ORIENTED_EDGE('',*,*,#1017,.T.);
#1329=ORIENTED_EDGE('',*,*,#1032,.T.);
#1330=ORIENTED_EDGE('',*,*,#1075,.F.);
#1331=ORIENTED_EDGE('',*,*,#1076,.F.);
#1332=ORIENTED_EDGE('',*,*,#977,.T.);
#1333=ORIENTED_EDGE('',*,*,#1077,.F.);
#1334=ORIENTED_EDGE('',*,*,#1078,.F.);
#1335=ORIENTED_EDGE('',*,*,#1062,.T.);
#1336=ORIENTED_EDGE('',*,*,#1018,.T.);
#1337=ORIENTED_EDGE('',*,*,#1076,.T.);
#1338=ORIENTED_EDGE('',*,*,#1079,.F.);
#1339=ORIENTED_EDGE('',*,*,#1080,.T.);
#1340=ORIENTED_EDGE('',*,*,#980,.T.);
#1341=ORIENTED_EDGE('',*,*,#1081,.T.);
#1342=ORIENTED_EDGE('',*,*,#1082,.T.);
#1343=ORIENTED_EDGE('',*,*,#1077,.T.);
#1344=ORIENTED_EDGE('',*,*,#1019,.T.);
#1345=ORIENTED_EDGE('',*,*,#1080,.F.);
#1346=ORIENTED_EDGE('',*,*,#1083,.F.);
#1347=ORIENTED_EDGE('',*,*,#1033,.F.);
#1348=ORIENTED_EDGE('',*,*,#979,.T.);
#1349=ORIENTED_EDGE('',*,*,#1061,.F.);
#1350=ORIENTED_EDGE('',*,*,#1084,.F.);
#1351=ORIENTED_EDGE('',*,*,#1081,.F.);
#1352=ORIENTED_EDGE('',*,*,#1013,.T.);
#1353=ORIENTED_EDGE('',*,*,#1035,.T.);
#1354=ORIENTED_EDGE('',*,*,#1085,.F.);
#1355=ORIENTED_EDGE('',*,*,#1086,.F.);
#1356=ORIENTED_EDGE('',*,*,#981,.T.);
#1357=ORIENTED_EDGE('',*,*,#1087,.F.);
#1358=ORIENTED_EDGE('',*,*,#1088,.F.);
#1359=ORIENTED_EDGE('',*,*,#1059,.T.);
#1360=ORIENTED_EDGE('',*,*,#1014,.T.);
#1361=ORIENTED_EDGE('',*,*,#1086,.T.);
#1362=ORIENTED_EDGE('',*,*,#1089,.F.);
#1363=ORIENTED_EDGE('',*,*,#1090,.T.);
#1364=ORIENTED_EDGE('',*,*,#984,.T.);
#1365=ORIENTED_EDGE('',*,*,#1091,.T.);
#1366=ORIENTED_EDGE('',*,*,#1092,.T.);
#1367=ORIENTED_EDGE('',*,*,#1087,.T.);
#1368=ORIENTED_EDGE('',*,*,#1015,.T.);
#1369=ORIENTED_EDGE('',*,*,#1090,.F.);
#1370=ORIENTED_EDGE('',*,*,#1093,.F.);
#1371=ORIENTED_EDGE('',*,*,#1036,.F.);
#1372=ORIENTED_EDGE('',*,*,#983,.T.);
#1373=ORIENTED_EDGE('',*,*,#1058,.F.);
#1374=ORIENTED_EDGE('',*,*,#1094,.F.);
#1375=ORIENTED_EDGE('',*,*,#1091,.F.);
#1376=ORIENTED_EDGE('',*,*,#1009,.T.);
#1377=ORIENTED_EDGE('',*,*,#1038,.T.);
#1378=ORIENTED_EDGE('',*,*,#1095,.F.);
#1379=ORIENTED_EDGE('',*,*,#1096,.F.);
#1380=ORIENTED_EDGE('',*,*,#985,.T.);
#1381=ORIENTED_EDGE('',*,*,#1097,.F.);
#1382=ORIENTED_EDGE('',*,*,#1098,.F.);
#1383=ORIENTED_EDGE('',*,*,#1056,.T.);
#1384=ORIENTED_EDGE('',*,*,#1010,.T.);
#1385=ORIENTED_EDGE('',*,*,#1096,.T.);
#1386=ORIENTED_EDGE('',*,*,#1099,.F.);
#1387=ORIENTED_EDGE('',*,*,#1100,.T.);
#1388=ORIENTED_EDGE('',*,*,#988,.T.);
#1389=ORIENTED_EDGE('',*,*,#1101,.T.);
#1390=ORIENTED_EDGE('',*,*,#1102,.T.);
#1391=ORIENTED_EDGE('',*,*,#1097,.T.);
#1392=ORIENTED_EDGE('',*,*,#1011,.T.);
#1393=ORIENTED_EDGE('',*,*,#1100,.F.);
#1394=ORIENTED_EDGE('',*,*,#1103,.F.);
#1395=ORIENTED_EDGE('',*,*,#1039,.F.);
#1396=ORIENTED_EDGE('',*,*,#987,.T.);
#1397=ORIENTED_EDGE('',*,*,#1055,.F.);
#1398=ORIENTED_EDGE('',*,*,#1104,.F.);
#1399=ORIENTED_EDGE('',*,*,#1101,.F.);
#1400=ORIENTED_EDGE('',*,*,#1005,.T.);
#1401=ORIENTED_EDGE('',*,*,#1041,.T.);
#1402=ORIENTED_EDGE('',*,*,#1105,.F.);
#1403=ORIENTED_EDGE('',*,*,#1106,.F.);
#1404=ORIENTED_EDGE('',*,*,#989,.T.);
#1405=ORIENTED_EDGE('',*,*,#1107,.F.);
#1406=ORIENTED_EDGE('',*,*,#1108,.F.);
#1407=ORIENTED_EDGE('',*,*,#1053,.T.);
#1408=ORIENTED_EDGE('',*,*,#1006,.T.);
#1409=ORIENTED_EDGE('',*,*,#1106,.T.);
#1410=ORIENTED_EDGE('',*,*,#1109,.F.);
#1411=ORIENTED_EDGE('',*,*,#1110,.T.);
#1412=ORIENTED_EDGE('',*,*,#992,.T.);
#1413=ORIENTED_EDGE('',*,*,#1111,.T.);
#1414=ORIENTED_EDGE('',*,*,#1112,.T.);
#1415=ORIENTED_EDGE('',*,*,#1107,.T.);
#1416=ORIENTED_EDGE('',*,*,#1007,.T.);
#1417=ORIENTED_EDGE('',*,*,#1110,.F.);
#1418=ORIENTED_EDGE('',*,*,#1113,.F.);
#1419=ORIENTED_EDGE('',*,*,#1042,.F.);
#1420=ORIENTED_EDGE('',*,*,#991,.T.);
#1421=ORIENTED_EDGE('',*,*,#1052,.F.);
#1422=ORIENTED_EDGE('',*,*,#1114,.F.);
#1423=ORIENTED_EDGE('',*,*,#1111,.F.);
#1424=ORIENTED_EDGE('',*,*,#1001,.T.);
#1425=ORIENTED_EDGE('',*,*,#1044,.T.);
#1426=ORIENTED_EDGE('',*,*,#1115,.F.);
#1427=ORIENTED_EDGE('',*,*,#1116,.F.);
#1428=ORIENTED_EDGE('',*,*,#993,.T.);
#1429=ORIENTED_EDGE('',*,*,#1117,.F.);
#1430=ORIENTED_EDGE('',*,*,#1118,.F.);
#1431=ORIENTED_EDGE('',*,*,#1050,.T.);
#1432=ORIENTED_EDGE('',*,*,#1002,.T.);
#1433=ORIENTED_EDGE('',*,*,#1116,.T.);
#1434=ORIENTED_EDGE('',*,*,#1119,.F.);
#1435=ORIENTED_EDGE('',*,*,#1120,.T.);
#1436=ORIENTED_EDGE('',*,*,#996,.T.);
#1437=ORIENTED_EDGE('',*,*,#1121,.T.);
#1438=ORIENTED_EDGE('',*,*,#1122,.T.);
#1439=ORIENTED_EDGE('',*,*,#1117,.T.);
#1440=ORIENTED_EDGE('',*,*,#1003,.T.);
#1441=ORIENTED_EDGE('',*,*,#1120,.F.);
#1442=ORIENTED_EDGE('',*,*,#1123,.F.);
#1443=ORIENTED_EDGE('',*,*,#1045,.F.);
#1444=ORIENTED_EDGE('',*,*,#995,.T.);
#1445=ORIENTED_EDGE('',*,*,#1049,.F.);
#1446=ORIENTED_EDGE('',*,*,#1124,.F.);
#1447=ORIENTED_EDGE('',*,*,#1121,.F.);
#1448=ORIENTED_EDGE('',*,*,#1074,.T.);
#1449=ORIENTED_EDGE('',*,*,#1063,.T.);
#1450=ORIENTED_EDGE('',*,*,#1078,.T.);
#1451=ORIENTED_EDGE('',*,*,#1082,.F.);
#1452=ORIENTED_EDGE('',*,*,#1084,.T.);
#1453=ORIENTED_EDGE('',*,*,#1060,.T.);
#1454=ORIENTED_EDGE('',*,*,#1088,.T.);
#1455=ORIENTED_EDGE('',*,*,#1092,.F.);
#1456=ORIENTED_EDGE('',*,*,#1094,.T.);
#1457=ORIENTED_EDGE('',*,*,#1057,.T.);
#1458=ORIENTED_EDGE('',*,*,#1098,.T.);
#1459=ORIENTED_EDGE('',*,*,#1102,.F.);
#1460=ORIENTED_EDGE('',*,*,#1104,.T.);
#1461=ORIENTED_EDGE('',*,*,#1054,.T.);
#1462=ORIENTED_EDGE('',*,*,#1108,.T.);
#1463=ORIENTED_EDGE('',*,*,#1112,.F.);
#1464=ORIENTED_EDGE('',*,*,#1114,.T.);
#1465=ORIENTED_EDGE('',*,*,#1051,.T.);
#1466=ORIENTED_EDGE('',*,*,#1118,.T.);
#1467=ORIENTED_EDGE('',*,*,#1122,.F.);
#1468=ORIENTED_EDGE('',*,*,#1124,.T.);
#1469=ORIENTED_EDGE('',*,*,#1048,.T.);
#1470=ORIENTED_EDGE('',*,*,#1125,.T.);
#1471=ORIENTED_EDGE('',*,*,#1126,.T.);
#1472=ORIENTED_EDGE('',*,*,#1127,.F.);
#1473=ORIENTED_EDGE('',*,*,#1026,.T.);
#1474=ORIENTED_EDGE('',*,*,#1068,.T.);
#1475=ORIENTED_EDGE('',*,*,#1072,.F.);
#1476=ORIENTED_EDGE('',*,*,#1047,.T.);
#1477=ORIENTED_EDGE('',*,*,#1128,.F.);
#1478=ORIENTED_EDGE('',*,*,#1129,.F.);
#1479=ORIENTED_EDGE('',*,*,#1125,.F.);
#1480=ORIENTED_EDGE('',*,*,#1073,.T.);
#1481=ORIENTED_EDGE('',*,*,#1069,.T.);
#1482=ORIENTED_EDGE('',*,*,#1065,.T.);
#1483=ORIENTED_EDGE('',*,*,#1028,.T.);
#1484=ORIENTED_EDGE('',*,*,#1130,.F.);
#1485=ORIENTED_EDGE('',*,*,#1131,.F.);
#1486=ORIENTED_EDGE('',*,*,#1128,.T.);
#1487=ORIENTED_EDGE('',*,*,#1046,.T.);
#1488=ORIENTED_EDGE('',*,*,#1123,.T.);
#1489=ORIENTED_EDGE('',*,*,#1119,.T.);
#1490=ORIENTED_EDGE('',*,*,#1115,.T.);
#1491=ORIENTED_EDGE('',*,*,#1043,.T.);
#1492=ORIENTED_EDGE('',*,*,#1113,.T.);
#1493=ORIENTED_EDGE('',*,*,#1109,.T.);
#1494=ORIENTED_EDGE('',*,*,#1105,.T.);
#1495=ORIENTED_EDGE('',*,*,#1040,.T.);
#1496=ORIENTED_EDGE('',*,*,#1103,.T.);
#1497=ORIENTED_EDGE('',*,*,#1099,.T.);
#1498=ORIENTED_EDGE('',*,*,#1095,.T.);
#1499=ORIENTED_EDGE('',*,*,#1037,.T.);
#1500=ORIENTED_EDGE('',*,*,#1093,.T.);
#1501=ORIENTED_EDGE('',*,*,#1089,.T.);
#1502=ORIENTED_EDGE('',*,*,#1085,.T.);
#1503=ORIENTED_EDGE('',*,*,#1034,.T.);
#1504=ORIENTED_EDGE('',*,*,#1083,.T.);
#1505=ORIENTED_EDGE('',*,*,#1079,.T.);
#1506=ORIENTED_EDGE('',*,*,#1075,.T.);
#1507=ORIENTED_EDGE('',*,*,#1031,.T.);
#1508=ORIENTED_EDGE('',*,*,#1129,.T.);
#1509=ORIENTED_EDGE('',*,*,#1131,.T.);
#1510=ORIENTED_EDGE('',*,*,#1132,.F.);
#1511=ORIENTED_EDGE('',*,*,#1126,.F.);
#1512=ORIENTED_EDGE('',*,*,#965,.T.);
#1513=ORIENTED_EDGE('',*,*,#968,.T.);
#1514=ORIENTED_EDGE('',*,*,#971,.T.);
#1515=ORIENTED_EDGE('',*,*,#974,.T.);
#1516=ORIENTED_EDGE('',*,*,#1027,.T.);
#1517=ORIENTED_EDGE('',*,*,#1127,.T.);
#1518=ORIENTED_EDGE('',*,*,#1132,.T.);
#1519=ORIENTED_EDGE('',*,*,#1130,.T.);
#1622=CYLINDRICAL_SURFACE('',#1777,0.409999999999997);
#1623=CYLINDRICAL_SURFACE('',#1781,0.409999999999997);
#1624=CYLINDRICAL_SURFACE('',#1785,0.409999999999997);
#1625=CYLINDRICAL_SURFACE('',#1789,0.409999999999997);
#1627=ADVANCED_FACE('',(#213),#1622,.F.);
#1628=ADVANCED_FACE('',(#214),#131,.F.);
#1629=ADVANCED_FACE('',(#215),#1623,.F.);
#1630=ADVANCED_FACE('',(#216),#132,.F.);
#1631=ADVANCED_FACE('',(#217),#1624,.F.);
#1632=ADVANCED_FACE('',(#218),#133,.F.);
#1633=ADVANCED_FACE('',(#219),#1625,.F.);
#1634=ADVANCED_FACE('',(#220),#134,.F.);
#1635=ADVANCED_FACE('',(#221),#135,.F.);
#1636=ADVANCED_FACE('',(#222),#136,.F.);
#1637=ADVANCED_FACE('',(#223),#137,.F.);
#1638=ADVANCED_FACE('',(#224),#138,.F.);
#1639=ADVANCED_FACE('',(#225),#139,.F.);
#1640=ADVANCED_FACE('',(#226),#140,.F.);
#1641=ADVANCED_FACE('',(#227),#141,.F.);
#1642=ADVANCED_FACE('',(#228),#142,.F.);
#1643=ADVANCED_FACE('',(#229),#143,.F.);
#1644=ADVANCED_FACE('',(#230),#144,.F.);
#1645=ADVANCED_FACE('',(#231),#145,.F.);
#1646=ADVANCED_FACE('',(#232),#146,.F.);
#1647=ADVANCED_FACE('',(#233),#147,.F.);
#1648=ADVANCED_FACE('',(#234),#148,.T.);
#1649=ADVANCED_FACE('',(#235),#149,.T.);
#1650=ADVANCED_FACE('',(#236),#150,.T.);
#1651=ADVANCED_FACE('',(#237),#151,.T.);
#1652=ADVANCED_FACE('',(#238),#152,.F.);
#1653=ADVANCED_FACE('',(#239),#153,.F.);
#1654=ADVANCED_FACE('',(#240),#154,.T.);
#1655=ADVANCED_FACE('',(#241),#155,.T.);
#1656=ADVANCED_FACE('',(#242),#156,.T.);
#1657=ADVANCED_FACE('',(#243),#157,.T.);
#1658=ADVANCED_FACE('',(#244),#158,.F.);
#1659=ADVANCED_FACE('',(#245),#159,.F.);
#1660=ADVANCED_FACE('',(#246),#160,.T.);
#1661=ADVANCED_FACE('',(#247),#161,.T.);
#1662=ADVANCED_FACE('',(#248),#162,.T.);
#1663=ADVANCED_FACE('',(#249),#163,.T.);
#1664=ADVANCED_FACE('',(#250),#164,.F.);
#1665=ADVANCED_FACE('',(#251),#165,.F.);
#1666=ADVANCED_FACE('',(#252),#166,.T.);
#1667=ADVANCED_FACE('',(#253),#167,.T.);
#1668=ADVANCED_FACE('',(#254),#168,.T.);
#1669=ADVANCED_FACE('',(#255),#169,.T.);
#1670=ADVANCED_FACE('',(#256),#170,.F.);
#1671=ADVANCED_FACE('',(#257),#171,.F.);
#1672=ADVANCED_FACE('',(#258),#172,.T.);
#1673=ADVANCED_FACE('',(#259),#173,.T.);
#1674=ADVANCED_FACE('',(#260),#174,.T.);
#1675=ADVANCED_FACE('',(#261),#175,.T.);
#1676=ADVANCED_FACE('',(#262),#176,.F.);
#1677=ADVANCED_FACE('',(#263),#177,.F.);
#1678=ADVANCED_FACE('',(#264),#178,.T.);
#1679=ADVANCED_FACE('',(#265),#179,.T.);
#1680=ADVANCED_FACE('',(#266),#180,.T.);
#1681=ADVANCED_FACE('',(#267),#181,.T.);
#1682=ADVANCED_FACE('',(#268),#182,.F.);
#1683=ADVANCED_FACE('',(#269),#183,.F.);
#1684=ADVANCED_FACE('',(#270),#184,.T.);
#1685=ADVANCED_FACE('',(#271),#185,.F.);
#1686=ADVANCED_FACE('',(#272),#186,.T.);
#1687=ADVANCED_FACE('',(#273,#127,#128,#129,#130),#187,.T.);
#1688=ADVANCED_FACE('',(#274),#188,.T.);
#1714=CLOSED_SHELL('',(#1627,#1628,#1629,#1630,#1631,#1632,#1633,#1634,
#1635,#1636,#1637,#1638,#1639,#1640,#1641,#1642,#1643,#1644,#1645,#1646,
#1647,#1648,#1649,#1650,#1651,#1652,#1653,#1654,#1655,#1656,#1657,#1658,
#1659,#1660,#1661,#1662,#1663,#1664,#1665,#1666,#1667,#1668,#1669,#1670,
#1671,#1672,#1673,#1674,#1675,#1676,#1677,#1678,#1679,#1680,#1681,#1682,
#1683,#1684,#1685,#1686,#1687,#1688));
#1776=AXIS2_PLACEMENT_3D('',#2366,#1904,#1905);
#1777=AXIS2_PLACEMENT_3D('',#2367,#1906,#1907);
#1778=AXIS2_PLACEMENT_3D('',#2369,#1908,#1909);
#1779=AXIS2_PLACEMENT_3D('',#2372,#1911,#1912);
#1780=AXIS2_PLACEMENT_3D('',#2373,#1913,#1914);
#1781=AXIS2_PLACEMENT_3D('',#2374,#1915,#1916);
#1782=AXIS2_PLACEMENT_3D('',#2376,#1917,#1918);
#1783=AXIS2_PLACEMENT_3D('',#2379,#1920,#1921);
#1784=AXIS2_PLACEMENT_3D('',#2380,#1922,#1923);
#1785=AXIS2_PLACEMENT_3D('',#2381,#1924,#1925);
#1786=AXIS2_PLACEMENT_3D('',#2383,#1926,#1927);
#1787=AXIS2_PLACEMENT_3D('',#2386,#1929,#1930);
#1788=AXIS2_PLACEMENT_3D('',#2387,#1931,#1932);
#1789=AXIS2_PLACEMENT_3D('',#2388,#1933,#1934);
#1790=AXIS2_PLACEMENT_3D('',#2390,#1935,#1936);
#1791=AXIS2_PLACEMENT_3D('',#2393,#1938,#1939);
#1792=AXIS2_PLACEMENT_3D('',#2394,#1940,#1941);
#1793=AXIS2_PLACEMENT_3D('',#2395,#1942,#1943);
#1794=AXIS2_PLACEMENT_3D('',#2404,#1948,#1949);
#1795=AXIS2_PLACEMENT_3D('',#2413,#1954,#1955);
#1796=AXIS2_PLACEMENT_3D('',#2422,#1960,#1961);
#1797=AXIS2_PLACEMENT_3D('',#2431,#1966,#1967);
#1798=AXIS2_PLACEMENT_3D('',#2440,#1972,#1973);
#1799=AXIS2_PLACEMENT_3D('',#2449,#1978,#1979);
#1800=AXIS2_PLACEMENT_3D('',#2458,#1984,#1985);
#1801=AXIS2_PLACEMENT_3D('',#2467,#1990,#1991);
#1802=AXIS2_PLACEMENT_3D('',#2476,#1996,#1997);
#1803=AXIS2_PLACEMENT_3D('',#2485,#2002,#2003);
#1804=AXIS2_PLACEMENT_3D('',#2494,#2008,#2009);
#1805=AXIS2_PLACEMENT_3D('',#2503,#2014,#2015);
#1806=AXIS2_PLACEMENT_3D('',#2572,#2056,#2057);
#1807=AXIS2_PLACEMENT_3D('',#2576,#2060,#2061);
#1808=AXIS2_PLACEMENT_3D('',#2580,#2064,#2065);
#1809=AXIS2_PLACEMENT_3D('',#2584,#2068,#2069);
#1810=AXIS2_PLACEMENT_3D('',#2588,#2072,#2073);
#1811=AXIS2_PLACEMENT_3D('',#2590,#2075,#2076);
#1812=AXIS2_PLACEMENT_3D('',#2592,#2078,#2079);
#1813=AXIS2_PLACEMENT_3D('',#2596,#2082,#2083);
#1814=AXIS2_PLACEMENT_3D('',#2600,#2086,#2087);
#1815=AXIS2_PLACEMENT_3D('',#2604,#2090,#2091);
#1816=AXIS2_PLACEMENT_3D('',#2608,#2094,#2095);
#1817=AXIS2_PLACEMENT_3D('',#2610,#2097,#2098);
#1818=AXIS2_PLACEMENT_3D('',#2612,#2100,#2101);
#1819=AXIS2_PLACEMENT_3D('',#2616,#2104,#2105);
#1820=AXIS2_PLACEMENT_3D('',#2620,#2108,#2109);
#1821=AXIS2_PLACEMENT_3D('',#2624,#2112,#2113);
#1822=AXIS2_PLACEMENT_3D('',#2628,#2116,#2117);
#1823=AXIS2_PLACEMENT_3D('',#2630,#2119,#2120);
#1824=AXIS2_PLACEMENT_3D('',#2632,#2122,#2123);
#1825=AXIS2_PLACEMENT_3D('',#2636,#2126,#2127);
#1826=AXIS2_PLACEMENT_3D('',#2640,#2130,#2131);
#1827=AXIS2_PLACEMENT_3D('',#2644,#2134,#2135);
#1828=AXIS2_PLACEMENT_3D('',#2648,#2138,#2139);
#1829=AXIS2_PLACEMENT_3D('',#2650,#2141,#2142);
#1830=AXIS2_PLACEMENT_3D('',#2652,#2144,#2145);
#1831=AXIS2_PLACEMENT_3D('',#2656,#2148,#2149);
#1832=AXIS2_PLACEMENT_3D('',#2660,#2152,#2153);
#1833=AXIS2_PLACEMENT_3D('',#2664,#2156,#2157);
#1834=AXIS2_PLACEMENT_3D('',#2668,#2160,#2161);
#1835=AXIS2_PLACEMENT_3D('',#2670,#2163,#2164);
#1836=AXIS2_PLACEMENT_3D('',#2672,#2166,#2167);
#1837=AXIS2_PLACEMENT_3D('',#2676,#2170,#2171);
#1838=AXIS2_PLACEMENT_3D('',#2680,#2174,#2175);
#1839=AXIS2_PLACEMENT_3D('',#2684,#2178,#2179);
#1840=AXIS2_PLACEMENT_3D('',#2688,#2182,#2183);
#1841=AXIS2_PLACEMENT_3D('',#2690,#2185,#2186);
#1842=AXIS2_PLACEMENT_3D('',#2692,#2188,#2189);
#1843=AXIS2_PLACEMENT_3D('',#2698,#2193,#2194);
#1844=AXIS2_PLACEMENT_3D('',#2702,#2197,#2198);
#1845=AXIS2_PLACEMENT_3D('',#2706,#2201,#2202);
#1846=AXIS2_PLACEMENT_3D('',#2708,#2204,#2205);
#1904=DIRECTION('axis',(0.,0.,1.));
#1905=DIRECTION('refdir',(1.,0.,0.));
#1906=DIRECTION('center_axis',(1.,0.,0.));
#1907=DIRECTION('ref_axis',(0.,0.,-1.));
#1908=DIRECTION('center_axis',(1.,0.,0.));
#1909=DIRECTION('ref_axis',(0.,0.,-1.));
#1910=DIRECTION('',(1.,0.,0.));
#1911=DIRECTION('center_axis',(1.,0.,0.));
#1912=DIRECTION('ref_axis',(0.,0.,-1.));
#1913=DIRECTION('center_axis',(1.,0.,0.));
#1914=DIRECTION('ref_axis',(0.,0.,-1.));
#1915=DIRECTION('center_axis',(1.,0.,0.));
#1916=DIRECTION('ref_axis',(0.,0.,-1.));
#1917=DIRECTION('center_axis',(1.,0.,0.));
#1918=DIRECTION('ref_axis',(0.,0.,-1.));
#1919=DIRECTION('',(1.,0.,0.));
#1920=DIRECTION('center_axis',(1.,0.,0.));
#1921=DIRECTION('ref_axis',(0.,0.,-1.));
#1922=DIRECTION('center_axis',(1.,0.,0.));
#1923=DIRECTION('ref_axis',(0.,0.,-1.));
#1924=DIRECTION('center_axis',(1.,0.,0.));
#1925=DIRECTION('ref_axis',(0.,0.,-1.));
#1926=DIRECTION('center_axis',(1.,0.,0.));
#1927=DIRECTION('ref_axis',(0.,0.,-1.));
#1928=DIRECTION('',(1.,0.,0.));
#1929=DIRECTION('center_axis',(1.,0.,0.));
#1930=DIRECTION('ref_axis',(0.,0.,-1.));
#1931=DIRECTION('center_axis',(1.,0.,0.));
#1932=DIRECTION('ref_axis',(0.,0.,-1.));
#1933=DIRECTION('center_axis',(1.,0.,0.));
#1934=DIRECTION('ref_axis',(0.,0.,-1.));
#1935=DIRECTION('center_axis',(1.,0.,0.));
#1936=DIRECTION('ref_axis',(0.,0.,-1.));
#1937=DIRECTION('',(1.,0.,0.));
#1938=DIRECTION('center_axis',(1.,0.,0.));
#1939=DIRECTION('ref_axis',(0.,0.,-1.));
#1940=DIRECTION('center_axis',(1.,0.,0.));
#1941=DIRECTION('ref_axis',(0.,0.,-1.));
#1942=DIRECTION('center_axis',(0.,1.,0.));
#1943=DIRECTION('ref_axis',(-1.,0.,0.));
#1944=DIRECTION('',(1.,0.,0.));
#1945=DIRECTION('',(0.,0.,1.));
#1946=DIRECTION('',(-1.,0.,0.));
#1947=DIRECTION('',(0.,0.,-1.));
#1948=DIRECTION('center_axis',(0.,1.,0.));
#1949=DIRECTION('ref_axis',(-1.,0.,0.));
#1950=DIRECTION('',(1.,0.,0.));
#1951=DIRECTION('',(0.,0.,1.));
#1952=DIRECTION('',(-1.,0.,0.));
#1953=DIRECTION('',(0.,0.,-1.));
#1954=DIRECTION('center_axis',(0.,1.,0.));
#1955=DIRECTION('ref_axis',(-1.,0.,0.));
#1956=DIRECTION('',(1.,0.,0.));
#1957=DIRECTION('',(0.,0.,1.));
#1958=DIRECTION('',(-1.,0.,0.));
#1959=DIRECTION('',(0.,0.,-1.));
#1960=DIRECTION('center_axis',(0.,1.,0.));
#1961=DIRECTION('ref_axis',(-1.,0.,0.));
#1962=DIRECTION('',(1.,0.,0.));
#1963=DIRECTION('',(0.,0.,1.));
#1964=DIRECTION('',(-1.,0.,0.));
#1965=DIRECTION('',(0.,0.,-1.));
#1966=DIRECTION('center_axis',(0.,1.,0.));
#1967=DIRECTION('ref_axis',(-1.,0.,0.));
#1968=DIRECTION('',(1.,0.,0.));
#1969=DIRECTION('',(0.,0.,1.));
#1970=DIRECTION('',(-1.,0.,0.));
#1971=DIRECTION('',(0.,0.,-1.));
#1972=DIRECTION('center_axis',(0.,1.,0.));
#1973=DIRECTION('ref_axis',(-1.,0.,0.));
#1974=DIRECTION('',(1.,0.,0.));
#1975=DIRECTION('',(0.,0.,1.));
#1976=DIRECTION('',(-1.,0.,0.));
#1977=DIRECTION('',(0.,0.,-1.));
#1978=DIRECTION('center_axis',(0.,-1.,0.));
#1979=DIRECTION('ref_axis',(1.,0.,0.));
#1980=DIRECTION('',(-1.,0.,0.));
#1981=DIRECTION('',(0.,0.,1.));
#1982=DIRECTION('',(1.,0.,0.));
#1983=DIRECTION('',(0.,0.,1.));
#1984=DIRECTION('center_axis',(0.,-1.,0.));
#1985=DIRECTION('ref_axis',(1.,0.,0.));
#1986=DIRECTION('',(-1.,0.,0.));
#1987=DIRECTION('',(0.,0.,1.));
#1988=DIRECTION('',(1.,0.,0.));
#1989=DIRECTION('',(0.,0.,1.));
#1990=DIRECTION('center_axis',(0.,-1.,0.));
#1991=DIRECTION('ref_axis',(1.,0.,0.));
#1992=DIRECTION('',(-1.,0.,0.));
#1993=DIRECTION('',(0.,0.,1.));
#1994=DIRECTION('',(1.,0.,0.));
#1995=DIRECTION('',(0.,0.,1.));
#1996=DIRECTION('center_axis',(0.,-1.,0.));
#1997=DIRECTION('ref_axis',(1.,0.,0.));
#1998=DIRECTION('',(-1.,0.,0.));
#1999=DIRECTION('',(0.,0.,1.));
#2000=DIRECTION('',(1.,0.,0.));
#2001=DIRECTION('',(0.,0.,1.));
#2002=DIRECTION('center_axis',(0.,-1.,0.));
#2003=DIRECTION('ref_axis',(1.,0.,0.));
#2004=DIRECTION('',(-1.,0.,0.));
#2005=DIRECTION('',(0.,0.,1.));
#2006=DIRECTION('',(1.,0.,0.));
#2007=DIRECTION('',(0.,0.,1.));
#2008=DIRECTION('center_axis',(0.,-1.,0.));
#2009=DIRECTION('ref_axis',(1.,0.,0.));
#2010=DIRECTION('',(-1.,0.,0.));
#2011=DIRECTION('',(0.,0.,1.));
#2012=DIRECTION('',(1.,0.,0.));
#2013=DIRECTION('',(0.,0.,1.));
#2014=DIRECTION('center_axis',(-1.,0.,0.));
#2015=DIRECTION('ref_axis',(0.,-1.,0.));
#2016=DIRECTION('',(0.,-1.,0.));
#2017=DIRECTION('',(0.,0.,-1.));
#2018=DIRECTION('',(0.,1.,0.));
#2019=DIRECTION('',(0.,0.,1.));
#2020=DIRECTION('',(0.,-1.,0.));
#2021=DIRECTION('',(0.,-1.,0.));
#2022=DIRECTION('',(0.,0.,1.));
#2023=DIRECTION('',(0.,-1.,0.));
#2024=DIRECTION('',(0.,-1.,0.));
#2025=DIRECTION('',(0.,0.,1.));
#2026=DIRECTION('',(0.,-1.,0.));
#2027=DIRECTION('',(0.,-1.,0.));
#2028=DIRECTION('',(0.,0.,1.));
#2029=DIRECTION('',(0.,-1.,0.));
#2030=DIRECTION('',(0.,-1.,0.));
#2031=DIRECTION('',(0.,0.,1.));
#2032=DIRECTION('',(0.,-1.,0.));
#2033=DIRECTION('',(0.,-1.,0.));
#2034=DIRECTION('',(0.,0.,1.));
#2035=DIRECTION('',(0.,-1.,0.));
#2036=DIRECTION('',(0.,-1.,0.));
#2037=DIRECTION('',(0.,0.,1.));
#2038=DIRECTION('',(0.,-1.,0.));
#2039=DIRECTION('',(0.,0.,-1.));
#2040=DIRECTION('',(0.,-1.,0.));
#2041=DIRECTION('',(0.,-1.,0.));
#2042=DIRECTION('',(0.,0.,-1.));
#2043=DIRECTION('',(0.,-1.,0.));
#2044=DIRECTION('',(0.,-1.,0.));
#2045=DIRECTION('',(0.,0.,-1.));
#2046=DIRECTION('',(0.,-1.,0.));
#2047=DIRECTION('',(0.,-1.,0.));
#2048=DIRECTION('',(0.,0.,-1.));
#2049=DIRECTION('',(0.,-1.,0.));
#2050=DIRECTION('',(0.,-1.,0.));
#2051=DIRECTION('',(0.,0.,-1.));
#2052=DIRECTION('',(0.,-1.,0.));
#2053=DIRECTION('',(0.,-1.,0.));
#2054=DIRECTION('',(0.,0.,-1.));
#2055=DIRECTION('',(0.,-1.,0.));
#2056=DIRECTION('center_axis',(0.,0.,1.));
#2057=DIRECTION('ref_axis',(1.,0.,0.));
#2058=DIRECTION('',(-1.,0.,0.));
#2059=DIRECTION('',(0.,-1.,0.));
#2060=DIRECTION('center_axis',(0.,0.,1.));
#2061=DIRECTION('ref_axis',(1.,0.,0.));
#2062=DIRECTION('',(0.,-1.,0.));
#2063=DIRECTION('',(1.,0.,0.));
#2064=DIRECTION('center_axis',(1.,0.,0.));
#2065=DIRECTION('ref_axis',(0.,1.,0.));
#2066=DIRECTION('',(0.,0.,1.));
#2067=DIRECTION('',(0.,1.,0.));
#2068=DIRECTION('center_axis',(1.,0.,0.));
#2069=DIRECTION('ref_axis',(0.,1.,0.));
#2070=DIRECTION('',(0.,1.,0.));
#2071=DIRECTION('',(0.,0.,1.));
#2072=DIRECTION('center_axis',(0.,0.,1.));
#2073=DIRECTION('ref_axis',(1.,0.,0.));
#2074=DIRECTION('',(1.,0.,0.));
#2075=DIRECTION('center_axis',(0.,0.,1.));
#2076=DIRECTION('ref_axis',(1.,0.,0.));
#2077=DIRECTION('',(-1.,0.,0.));
#2078=DIRECTION('center_axis',(0.,0.,1.));
#2079=DIRECTION('ref_axis',(1.,0.,0.));
#2080=DIRECTION('',(-1.,0.,0.));
#2081=DIRECTION('',(0.,-1.,0.));
#2082=DIRECTION('center_axis',(0.,0.,1.));
#2083=DIRECTION('ref_axis',(1.,0.,0.));
#2084=DIRECTION('',(0.,-1.,0.));
#2085=DIRECTION('',(1.,0.,0.));
#2086=DIRECTION('center_axis',(1.,0.,0.));
#2087=DIRECTION('ref_axis',(0.,1.,0.));
#2088=DIRECTION('',(0.,0.,1.));
#2089=DIRECTION('',(0.,1.,0.));
#2090=DIRECTION('center_axis',(1.,0.,0.));
#2091=DIRECTION('ref_axis',(0.,1.,0.));
#2092=DIRECTION('',(0.,1.,0.));
#2093=DIRECTION('',(0.,0.,1.));
#2094=DIRECTION('center_axis',(0.,0.,1.));
#2095=DIRECTION('ref_axis',(1.,0.,0.));
#2096=DIRECTION('',(1.,0.,0.));
#2097=DIRECTION('center_axis',(0.,0.,1.));
#2098=DIRECTION('ref_axis',(1.,0.,0.));
#2099=DIRECTION('',(-1.,0.,0.));
#2100=DIRECTION('center_axis',(0.,0.,1.));
#2101=DIRECTION('ref_axis',(1.,0.,0.));
#2102=DIRECTION('',(-1.,0.,0.));
#2103=DIRECTION('',(0.,-1.,0.));
#2104=DIRECTION('center_axis',(0.,0.,1.));
#2105=DIRECTION('ref_axis',(1.,0.,0.));
#2106=DIRECTION('',(0.,-1.,0.));
#2107=DIRECTION('',(1.,0.,0.));
#2108=DIRECTION('center_axis',(1.,0.,0.));
#2109=DIRECTION('ref_axis',(0.,1.,0.));
#2110=DIRECTION('',(0.,0.,1.));
#2111=DIRECTION('',(0.,1.,0.));
#2112=DIRECTION('center_axis',(1.,0.,0.));
#2113=DIRECTION('ref_axis',(0.,1.,0.));
#2114=DIRECTION('',(0.,1.,0.));
#2115=DIRECTION('',(0.,0.,1.));
#2116=DIRECTION('center_axis',(0.,0.,1.));
#2117=DIRECTION('ref_axis',(1.,0.,0.));
#2118=DIRECTION('',(1.,0.,0.));
#2119=DIRECTION('center_axis',(0.,0.,1.));
#2120=DIRECTION('ref_axis',(1.,0.,0.));
#2121=DIRECTION('',(-1.,0.,0.));
#2122=DIRECTION('center_axis',(0.,0.,1.));
#2123=DIRECTION('ref_axis',(1.,0.,0.));
#2124=DIRECTION('',(-1.,0.,0.));
#2125=DIRECTION('',(0.,-1.,0.));
#2126=DIRECTION('center_axis',(0.,0.,1.));
#2127=DIRECTION('ref_axis',(1.,0.,0.));
#2128=DIRECTION('',(0.,-1.,0.));
#2129=DIRECTION('',(1.,0.,0.));
#2130=DIRECTION('center_axis',(1.,0.,0.));
#2131=DIRECTION('ref_axis',(0.,1.,0.));
#2132=DIRECTION('',(0.,0.,1.));
#2133=DIRECTION('',(0.,1.,0.));
#2134=DIRECTION('center_axis',(1.,0.,0.));
#2135=DIRECTION('ref_axis',(0.,1.,0.));
#2136=DIRECTION('',(0.,1.,0.));
#2137=DIRECTION('',(0.,0.,1.));
#2138=DIRECTION('center_axis',(0.,0.,1.));
#2139=DIRECTION('ref_axis',(1.,0.,0.));
#2140=DIRECTION('',(1.,0.,0.));
#2141=DIRECTION('center_axis',(0.,0.,1.));
#2142=DIRECTION('ref_axis',(1.,0.,0.));
#2143=DIRECTION('',(-1.,0.,0.));
#2144=DIRECTION('center_axis',(0.,0.,1.));
#2145=DIRECTION('ref_axis',(1.,0.,0.));
#2146=DIRECTION('',(-1.,0.,0.));
#2147=DIRECTION('',(0.,-1.,0.));
#2148=DIRECTION('center_axis',(0.,0.,1.));
#2149=DIRECTION('ref_axis',(1.,0.,0.));
#2150=DIRECTION('',(0.,-1.,0.));
#2151=DIRECTION('',(1.,0.,0.));
#2152=DIRECTION('center_axis',(1.,0.,0.));
#2153=DIRECTION('ref_axis',(0.,1.,0.));
#2154=DIRECTION('',(0.,0.,1.));
#2155=DIRECTION('',(0.,1.,0.));
#2156=DIRECTION('center_axis',(1.,0.,0.));
#2157=DIRECTION('ref_axis',(0.,1.,0.));
#2158=DIRECTION('',(0.,1.,0.));
#2159=DIRECTION('',(0.,0.,1.));
#2160=DIRECTION('center_axis',(0.,0.,1.));
#2161=DIRECTION('ref_axis',(1.,0.,0.));
#2162=DIRECTION('',(1.,0.,0.));
#2163=DIRECTION('center_axis',(0.,0.,1.));
#2164=DIRECTION('ref_axis',(1.,0.,0.));
#2165=DIRECTION('',(-1.,0.,0.));
#2166=DIRECTION('center_axis',(0.,0.,1.));
#2167=DIRECTION('ref_axis',(1.,0.,0.));
#2168=DIRECTION('',(-1.,0.,0.));
#2169=DIRECTION('',(0.,-1.,0.));
#2170=DIRECTION('center_axis',(0.,0.,1.));
#2171=DIRECTION('ref_axis',(1.,0.,0.));
#2172=DIRECTION('',(0.,-1.,0.));
#2173=DIRECTION('',(1.,0.,0.));
#2174=DIRECTION('center_axis',(1.,0.,0.));
#2175=DIRECTION('ref_axis',(0.,1.,0.));
#2176=DIRECTION('',(0.,0.,1.));
#2177=DIRECTION('',(0.,1.,0.));
#2178=DIRECTION('center_axis',(1.,0.,0.));
#2179=DIRECTION('ref_axis',(0.,1.,0.));
#2180=DIRECTION('',(0.,1.,0.));
#2181=DIRECTION('',(0.,0.,1.));
#2182=DIRECTION('center_axis',(0.,0.,1.));
#2183=DIRECTION('ref_axis',(1.,0.,0.));
#2184=DIRECTION('',(1.,0.,0.));
#2185=DIRECTION('center_axis',(0.,0.,1.));
#2186=DIRECTION('ref_axis',(1.,0.,0.));
#2187=DIRECTION('',(-1.,0.,0.));
#2188=DIRECTION('center_axis',(0.,1.,0.));
#2189=DIRECTION('ref_axis',(-1.,0.,0.));
#2190=DIRECTION('',(-1.,0.,0.));
#2191=DIRECTION('',(0.,0.,1.));
#2192=DIRECTION('',(-1.,0.,0.));
#2193=DIRECTION('center_axis',(0.,0.,1.));
#2194=DIRECTION('ref_axis',(1.,0.,0.));
#2195=DIRECTION('',(1.,0.,0.));
#2196=DIRECTION('',(0.,-1.,0.));
#2197=DIRECTION('center_axis',(0.,-1.,0.));
#2198=DIRECTION('ref_axis',(1.,0.,0.));
#2199=DIRECTION('',(1.,0.,0.));
#2200=DIRECTION('',(0.,0.,1.));
#2201=DIRECTION('center_axis',(-1.,0.,0.));
#2202=DIRECTION('ref_axis',(0.,-1.,0.));
#2203=DIRECTION('',(0.,-1.,0.));
#2204=DIRECTION('center_axis',(0.,0.,1.));
#2205=DIRECTION('ref_axis',(1.,0.,0.));
#2366=CARTESIAN_POINT('',(0.,0.,0.));
#2367=CARTESIAN_POINT('Origin',(0.,51.,64.));
#2368=CARTESIAN_POINT('',(0.,51.,64.41));
#2369=CARTESIAN_POINT('Origin',(0.,51.,64.));
#2370=CARTESIAN_POINT('',(1.5,51.,64.41));
#2371=CARTESIAN_POINT('',(0.,51.,64.41));
#2372=CARTESIAN_POINT('Origin',(1.5,51.,64.));
#2373=CARTESIAN_POINT('Origin',(1.5,51.,64.));
#2374=CARTESIAN_POINT('Origin',(0.,9.,116.));
#2375=CARTESIAN_POINT('',(0.,9.,116.41));
#2376=CARTESIAN_POINT('Origin',(0.,9.,116.));
#2377=CARTESIAN_POINT('',(1.5,9.,116.41));
#2378=CARTESIAN_POINT('',(0.,9.,116.41));
#2379=CARTESIAN_POINT('Origin',(1.5,9.,116.));
#2380=CARTESIAN_POINT('Origin',(1.5,9.,116.));
#2381=CARTESIAN_POINT('Origin',(0.,9.,64.));
#2382=CARTESIAN_POINT('',(0.,9.,64.41));
#2383=CARTESIAN_POINT('Origin',(0.,9.,64.));
#2384=CARTESIAN_POINT('',(1.5,9.,64.41));
#2385=CARTESIAN_POINT('',(0.,9.,64.41));
#2386=CARTESIAN_POINT('Origin',(1.5,9.,64.));
#2387=CARTESIAN_POINT('Origin',(1.5,9.,64.));
#2388=CARTESIAN_POINT('Origin',(0.,51.,116.));
#2389=CARTESIAN_POINT('',(0.,51.,116.41));
#2390=CARTESIAN_POINT('Origin',(0.,51.,116.));
#2391=CARTESIAN_POINT('',(1.5,51.,116.41));
#2392=CARTESIAN_POINT('',(0.,51.,116.41));
#2393=CARTESIAN_POINT('Origin',(1.5,51.,116.));
#2394=CARTESIAN_POINT('Origin',(1.5,51.,116.));
#2395=CARTESIAN_POINT('Origin',(1.81,58.82,0.));
#2396=CARTESIAN_POINT('',(1.3,58.82,149.08));
#2397=CARTESIAN_POINT('',(1.8,58.82,149.08));
#2398=CARTESIAN_POINT('',(1.6825,58.82,149.08));
#2399=CARTESIAN_POINT('',(1.3,58.82,120.92));
#2400=CARTESIAN_POINT('',(1.3,58.82,0.));
#2401=CARTESIAN_POINT('',(1.8,58.82,120.92));
#2402=CARTESIAN_POINT('',(1.6825,58.82,120.92));
#2403=CARTESIAN_POINT('',(1.8,58.82,0.));
#2404=CARTESIAN_POINT('Origin',(1.81,58.82,0.));
#2405=CARTESIAN_POINT('',(1.3,58.82,119.08));
#2406=CARTESIAN_POINT('',(1.8,58.82,119.08));
#2407=CARTESIAN_POINT('',(1.6825,58.82,119.08));
#2408=CARTESIAN_POINT('',(1.3,58.82,90.92));
#2409=CARTESIAN_POINT('',(1.3,58.82,0.));
#2410=CARTESIAN_POINT('',(1.8,58.82,90.92));
#2411=CARTESIAN_POINT('',(1.6825,58.82,90.92));
#2412=CARTESIAN_POINT('',(1.8,58.82,0.));
#2413=CARTESIAN_POINT('Origin',(1.81,58.82,0.));
#2414=CARTESIAN_POINT('',(1.3,58.82,89.08));
#2415=CARTESIAN_POINT('',(1.8,58.82,89.08));
#2416=CARTESIAN_POINT('',(1.6825,58.82,89.08));
#2417=CARTESIAN_POINT('',(1.3,58.82,60.92));
#2418=CARTESIAN_POINT('',(1.3,58.82,0.));
#2419=CARTESIAN_POINT('',(1.8,58.82,60.92));
#2420=CARTESIAN_POINT('',(1.6825,58.82,60.92));
#2421=CARTESIAN_POINT('',(1.8,58.82,0.));
#2422=CARTESIAN_POINT('Origin',(1.81,58.82,0.));
#2423=CARTESIAN_POINT('',(1.3,58.82,59.08));
#2424=CARTESIAN_POINT('',(1.8,58.82,59.08));
#2425=CARTESIAN_POINT('',(1.6825,58.82,59.08));
#2426=CARTESIAN_POINT('',(1.3,58.82,30.92));
#2427=CARTESIAN_POINT('',(1.3,58.82,0.));
#2428=CARTESIAN_POINT('',(1.8,58.82,30.92));
#2429=CARTESIAN_POINT('',(1.6825,58.82,30.92));
#2430=CARTESIAN_POINT('',(1.8,58.82,0.));
#2431=CARTESIAN_POINT('Origin',(1.81,58.82,0.));
#2432=CARTESIAN_POINT('',(1.3,58.82,29.08));
#2433=CARTESIAN_POINT('',(1.8,58.82,29.08));
#2434=CARTESIAN_POINT('',(1.6825,58.82,29.08));
#2435=CARTESIAN_POINT('',(1.3,58.82,1.82));
#2436=CARTESIAN_POINT('',(1.3,58.82,0.));
#2437=CARTESIAN_POINT('',(1.8,58.82,1.82));
#2438=CARTESIAN_POINT('',(1.6825,58.82,1.82));
#2439=CARTESIAN_POINT('',(1.8,58.82,0.));
#2440=CARTESIAN_POINT('Origin',(1.81,58.82,0.));
#2441=CARTESIAN_POINT('',(1.3,58.82,178.18));
#2442=CARTESIAN_POINT('',(1.8,58.82,178.18));
#2443=CARTESIAN_POINT('',(1.6825,58.82,178.18));
#2444=CARTESIAN_POINT('',(1.3,58.82,150.92));
#2445=CARTESIAN_POINT('',(1.3,58.82,0.));
#2446=CARTESIAN_POINT('',(1.8,58.82,150.92));
#2447=CARTESIAN_POINT('',(1.6825,58.82,150.92));
#2448=CARTESIAN_POINT('',(1.8,58.82,0.));
#2449=CARTESIAN_POINT('Origin',(1.3,58.18,0.));
#2450=CARTESIAN_POINT('',(1.8,58.18,29.08));
#2451=CARTESIAN_POINT('',(1.3,58.18,29.08));
#2452=CARTESIAN_POINT('',(1.4275,58.18,29.08));
#2453=CARTESIAN_POINT('',(1.8,58.18,1.82));
#2454=CARTESIAN_POINT('',(1.8,58.18,0.));
#2455=CARTESIAN_POINT('',(1.3,58.18,1.82));
#2456=CARTESIAN_POINT('',(1.4275,58.18,1.82));
#2457=CARTESIAN_POINT('',(1.3,58.18,0.));
#2458=CARTESIAN_POINT('Origin',(1.3,58.18,0.));
#2459=CARTESIAN_POINT('',(1.8,58.18,59.08));
#2460=CARTESIAN_POINT('',(1.3,58.18,59.08));
#2461=CARTESIAN_POINT('',(1.4275,58.18,59.08));
#2462=CARTESIAN_POINT('',(1.8,58.18,30.92));
#2463=CARTESIAN_POINT('',(1.8,58.18,0.));
#2464=CARTESIAN_POINT('',(1.3,58.18,30.92));
#2465=CARTESIAN_POINT('',(1.4275,58.18,30.92));
#2466=CARTESIAN_POINT('',(1.3,58.18,0.));
#2467=CARTESIAN_POINT('Origin',(1.3,58.18,0.));
#2468=CARTESIAN_POINT('',(1.8,58.18,89.08));
#2469=CARTESIAN_POINT('',(1.3,58.18,89.08));
#2470=CARTESIAN_POINT('',(1.4275,58.18,89.08));
#2471=CARTESIAN_POINT('',(1.8,58.18,60.92));
#2472=CARTESIAN_POINT('',(1.8,58.18,0.));
#2473=CARTESIAN_POINT('',(1.3,58.18,60.92));
#2474=CARTESIAN_POINT('',(1.4275,58.18,60.92));
#2475=CARTESIAN_POINT('',(1.3,58.18,0.));
#2476=CARTESIAN_POINT('Origin',(1.3,58.18,0.));
#2477=CARTESIAN_POINT('',(1.8,58.18,119.08));
#2478=CARTESIAN_POINT('',(1.3,58.18,119.08));
#2479=CARTESIAN_POINT('',(1.4275,58.18,119.08));
#2480=CARTESIAN_POINT('',(1.8,58.18,90.92));
#2481=CARTESIAN_POINT('',(1.8,58.18,0.));
#2482=CARTESIAN_POINT('',(1.3,58.18,90.92));
#2483=CARTESIAN_POINT('',(1.4275,58.18,90.92));
#2484=CARTESIAN_POINT('',(1.3,58.18,0.));
#2485=CARTESIAN_POINT('Origin',(1.3,58.18,0.));
#2486=CARTESIAN_POINT('',(1.8,58.18,149.08));
#2487=CARTESIAN_POINT('',(1.3,58.18,149.08));
#2488=CARTESIAN_POINT('',(1.4275,58.18,149.08));
#2489=CARTESIAN_POINT('',(1.8,58.18,120.92));
#2490=CARTESIAN_POINT('',(1.8,58.18,0.));
#2491=CARTESIAN_POINT('',(1.3,58.18,120.92));
#2492=CARTESIAN_POINT('',(1.4275,58.18,120.92));
#2493=CARTESIAN_POINT('',(1.3,58.18,0.));
#2494=CARTESIAN_POINT('Origin',(1.3,58.18,0.));
#2495=CARTESIAN_POINT('',(1.8,58.18,178.18));
#2496=CARTESIAN_POINT('',(1.3,58.18,178.18));
#2497=CARTESIAN_POINT('',(1.4275,58.18,178.18));
#2498=CARTESIAN_POINT('',(1.8,58.18,150.92));
#2499=CARTESIAN_POINT('',(1.8,58.18,0.));
#2500=CARTESIAN_POINT('',(1.3,58.18,150.92));
#2501=CARTESIAN_POINT('',(1.4275,58.18,150.92));
#2502=CARTESIAN_POINT('',(1.3,58.18,0.));
#2503=CARTESIAN_POINT('Origin',(1.3,60.,178.18));
#2504=CARTESIAN_POINT('',(1.3,60.,178.18));
#2505=CARTESIAN_POINT('',(1.3,60.,178.18));
#2506=CARTESIAN_POINT('',(1.3,60.,180.));
#2507=CARTESIAN_POINT('',(1.3,60.,89.09));
#2508=CARTESIAN_POINT('',(1.3,0.,180.));
#2509=CARTESIAN_POINT('',(1.3,45.,180.));
#2510=CARTESIAN_POINT('',(1.3,0.,178.18));
#2511=CARTESIAN_POINT('',(1.3,0.,89.09));
#2512=CARTESIAN_POINT('',(1.3,60.,178.18));
#2513=CARTESIAN_POINT('',(1.3,0.,150.92));
#2514=CARTESIAN_POINT('',(1.3,60.,150.92));
#2515=CARTESIAN_POINT('',(1.3,0.,149.08));
#2516=CARTESIAN_POINT('',(1.3,0.,74.54));
#2517=CARTESIAN_POINT('',(1.3,60.,149.08));
#2518=CARTESIAN_POINT('',(1.3,0.,120.92));
#2519=CARTESIAN_POINT('',(1.3,60.,120.92));
#2520=CARTESIAN_POINT('',(1.3,0.,119.08));
#2521=CARTESIAN_POINT('',(1.3,0.,59.54));
#2522=CARTESIAN_POINT('',(1.3,60.,119.08));
#2523=CARTESIAN_POINT('',(1.3,0.,90.92));
#2524=CARTESIAN_POINT('',(1.3,60.,90.92));
#2525=CARTESIAN_POINT('',(1.3,0.,89.08));
#2526=CARTESIAN_POINT('',(1.3,0.,44.54));
#2527=CARTESIAN_POINT('',(1.3,60.,89.08));
#2528=CARTESIAN_POINT('',(1.3,0.,60.92));
#2529=CARTESIAN_POINT('',(1.3,60.,60.92));
#2530=CARTESIAN_POINT('',(1.3,0.,59.08));
#2531=CARTESIAN_POINT('',(1.3,0.,29.54));
#2532=CARTESIAN_POINT('',(1.3,60.,59.08));
#2533=CARTESIAN_POINT('',(1.3,0.,30.92));
#2534=CARTESIAN_POINT('',(1.3,60.,30.92));
#2535=CARTESIAN_POINT('',(1.3,0.,29.08));
#2536=CARTESIAN_POINT('',(1.3,0.,14.54));
#2537=CARTESIAN_POINT('',(1.3,60.,29.08));
#2538=CARTESIAN_POINT('',(1.3,0.,1.82));
#2539=CARTESIAN_POINT('',(1.3,60.,1.82));
#2540=CARTESIAN_POINT('',(1.3,0.,0.));
#2541=CARTESIAN_POINT('',(1.3,0.,0.));
#2542=CARTESIAN_POINT('',(1.3,60.,0.));
#2543=CARTESIAN_POINT('',(1.3,45.,0.));
#2544=CARTESIAN_POINT('',(1.3,60.,1.82));
#2545=CARTESIAN_POINT('',(1.3,60.,0.));
#2546=CARTESIAN_POINT('',(1.3,60.,1.82));
#2547=CARTESIAN_POINT('',(1.3,60.,29.08));
#2548=CARTESIAN_POINT('',(1.3,60.,29.08));
#2549=CARTESIAN_POINT('',(1.3,60.,30.92));
#2550=CARTESIAN_POINT('',(1.3,60.,14.54));
#2551=CARTESIAN_POINT('',(1.3,60.,30.92));
#2552=CARTESIAN_POINT('',(1.3,60.,59.08));
#2553=CARTESIAN_POINT('',(1.3,60.,59.08));
#2554=CARTESIAN_POINT('',(1.3,60.,60.92));
#2555=CARTESIAN_POINT('',(1.3,60.,29.54));
#2556=CARTESIAN_POINT('',(1.3,60.,60.92));
#2557=CARTESIAN_POINT('',(1.3,60.,89.08));
#2558=CARTESIAN_POINT('',(1.3,60.,89.08));
#2559=CARTESIAN_POINT('',(1.3,60.,90.92));
#2560=CARTESIAN_POINT('',(1.3,60.,44.54));
#2561=CARTESIAN_POINT('',(1.3,60.,90.92));
#2562=CARTESIAN_POINT('',(1.3,60.,119.08));
#2563=CARTESIAN_POINT('',(1.3,60.,119.08));
#2564=CARTESIAN_POINT('',(1.3,60.,120.92));
#2565=CARTESIAN_POINT('',(1.3,60.,59.54));
#2566=CARTESIAN_POINT('',(1.3,60.,120.92));
#2567=CARTESIAN_POINT('',(1.3,60.,149.08));
#2568=CARTESIAN_POINT('',(1.3,60.,149.08));
#2569=CARTESIAN_POINT('',(1.3,60.,150.92));
#2570=CARTESIAN_POINT('',(1.3,60.,74.54));
#2571=CARTESIAN_POINT('',(1.3,60.,150.92));
#2572=CARTESIAN_POINT('Origin',(1.555,30.,178.18));
#2573=CARTESIAN_POINT('',(1.8,0.,178.18));
#2574=CARTESIAN_POINT('',(0.7775,0.,178.18));
#2575=CARTESIAN_POINT('',(1.8,15.,178.18));
#2576=CARTESIAN_POINT('Origin',(1.555,30.,178.18));
#2577=CARTESIAN_POINT('',(1.8,60.,178.18));
#2578=CARTESIAN_POINT('',(1.8,15.,178.18));
#2579=CARTESIAN_POINT('',(1.6775,60.,178.18));
#2580=CARTESIAN_POINT('Origin',(1.8,0.,0.));
#2581=CARTESIAN_POINT('',(1.8,0.,150.92));
#2582=CARTESIAN_POINT('',(1.8,0.,0.));
#2583=CARTESIAN_POINT('',(1.8,15.,150.92));
#2584=CARTESIAN_POINT('Origin',(1.8,0.,0.));
#2585=CARTESIAN_POINT('',(1.8,60.,150.92));
#2586=CARTESIAN_POINT('',(1.8,15.,150.92));
#2587=CARTESIAN_POINT('',(1.8,60.,0.));
#2588=CARTESIAN_POINT('Origin',(1.555,30.,150.92));
#2589=CARTESIAN_POINT('',(0.7775,0.,150.92));
#2590=CARTESIAN_POINT('Origin',(1.555,30.,150.92));
#2591=CARTESIAN_POINT('',(1.6775,60.,150.92));
#2592=CARTESIAN_POINT('Origin',(1.555,30.,149.08));
#2593=CARTESIAN_POINT('',(1.8,0.,149.08));
#2594=CARTESIAN_POINT('',(0.7775,0.,149.08));
#2595=CARTESIAN_POINT('',(1.8,15.,149.08));
#2596=CARTESIAN_POINT('Origin',(1.555,30.,149.08));
#2597=CARTESIAN_POINT('',(1.8,60.,149.08));
#2598=CARTESIAN_POINT('',(1.8,15.,149.08));
#2599=CARTESIAN_POINT('',(1.6775,60.,149.08));
#2600=CARTESIAN_POINT('Origin',(1.8,0.,0.));
#2601=CARTESIAN_POINT('',(1.8,0.,120.92));
#2602=CARTESIAN_POINT('',(1.8,0.,0.));
#2603=CARTESIAN_POINT('',(1.8,15.,120.92));
#2604=CARTESIAN_POINT('Origin',(1.8,0.,0.));
#2605=CARTESIAN_POINT('',(1.8,60.,120.92));
#2606=CARTESIAN_POINT('',(1.8,15.,120.92));
#2607=CARTESIAN_POINT('',(1.8,60.,0.));
#2608=CARTESIAN_POINT('Origin',(1.555,30.,120.92));
#2609=CARTESIAN_POINT('',(0.7775,0.,120.92));
#2610=CARTESIAN_POINT('Origin',(1.555,30.,120.92));
#2611=CARTESIAN_POINT('',(1.6775,60.,120.92));
#2612=CARTESIAN_POINT('Origin',(1.555,30.,119.08));
#2613=CARTESIAN_POINT('',(1.8,0.,119.08));
#2614=CARTESIAN_POINT('',(0.7775,0.,119.08));
#2615=CARTESIAN_POINT('',(1.8,15.,119.08));
#2616=CARTESIAN_POINT('Origin',(1.555,30.,119.08));
#2617=CARTESIAN_POINT('',(1.8,60.,119.08));
#2618=CARTESIAN_POINT('',(1.8,15.,119.08));
#2619=CARTESIAN_POINT('',(1.6775,60.,119.08));
#2620=CARTESIAN_POINT('Origin',(1.8,0.,0.));
#2621=CARTESIAN_POINT('',(1.8,0.,90.92));
#2622=CARTESIAN_POINT('',(1.8,0.,0.));
#2623=CARTESIAN_POINT('',(1.8,15.,90.92));
#2624=CARTESIAN_POINT('Origin',(1.8,0.,0.));
#2625=CARTESIAN_POINT('',(1.8,60.,90.92));
#2626=CARTESIAN_POINT('',(1.8,15.,90.92));
#2627=CARTESIAN_POINT('',(1.8,60.,0.));
#2628=CARTESIAN_POINT('Origin',(1.555,30.,90.92));
#2629=CARTESIAN_POINT('',(0.7775,0.,90.92));
#2630=CARTESIAN_POINT('Origin',(1.555,30.,90.92));
#2631=CARTESIAN_POINT('',(1.6775,60.,90.92));
#2632=CARTESIAN_POINT('Origin',(1.555,30.,89.08));
#2633=CARTESIAN_POINT('',(1.8,0.,89.08));
#2634=CARTESIAN_POINT('',(0.7775,0.,89.08));
#2635=CARTESIAN_POINT('',(1.8,15.,89.08));
#2636=CARTESIAN_POINT('Origin',(1.555,30.,89.08));
#2637=CARTESIAN_POINT('',(1.8,60.,89.08));
#2638=CARTESIAN_POINT('',(1.8,15.,89.08));
#2639=CARTESIAN_POINT('',(1.6775,60.,89.08));
#2640=CARTESIAN_POINT('Origin',(1.8,0.,0.));
#2641=CARTESIAN_POINT('',(1.8,0.,60.92));
#2642=CARTESIAN_POINT('',(1.8,0.,0.));
#2643=CARTESIAN_POINT('',(1.8,15.,60.92));
#2644=CARTESIAN_POINT('Origin',(1.8,0.,0.));
#2645=CARTESIAN_POINT('',(1.8,60.,60.92));
#2646=CARTESIAN_POINT('',(1.8,15.,60.92));
#2647=CARTESIAN_POINT('',(1.8,60.,0.));
#2648=CARTESIAN_POINT('Origin',(1.555,30.,60.92));
#2649=CARTESIAN_POINT('',(0.7775,0.,60.92));
#2650=CARTESIAN_POINT('Origin',(1.555,30.,60.92));
#2651=CARTESIAN_POINT('',(1.6775,60.,60.92));
#2652=CARTESIAN_POINT('Origin',(1.555,30.,59.08));
#2653=CARTESIAN_POINT('',(1.8,0.,59.08));
#2654=CARTESIAN_POINT('',(0.7775,0.,59.08));
#2655=CARTESIAN_POINT('',(1.8,15.,59.08));
#2656=CARTESIAN_POINT('Origin',(1.555,30.,59.08));
#2657=CARTESIAN_POINT('',(1.8,60.,59.08));
#2658=CARTESIAN_POINT('',(1.8,15.,59.08));
#2659=CARTESIAN_POINT('',(1.6775,60.,59.08));
#2660=CARTESIAN_POINT('Origin',(1.8,0.,0.));
#2661=CARTESIAN_POINT('',(1.8,0.,30.92));
#2662=CARTESIAN_POINT('',(1.8,0.,0.));
#2663=CARTESIAN_POINT('',(1.8,15.,30.92));
#2664=CARTESIAN_POINT('Origin',(1.8,0.,0.));
#2665=CARTESIAN_POINT('',(1.8,60.,30.92));
#2666=CARTESIAN_POINT('',(1.8,15.,30.92));
#2667=CARTESIAN_POINT('',(1.8,60.,0.));
#2668=CARTESIAN_POINT('Origin',(1.555,30.,30.92));
#2669=CARTESIAN_POINT('',(0.7775,0.,30.92));
#2670=CARTESIAN_POINT('Origin',(1.555,30.,30.92));
#2671=CARTESIAN_POINT('',(1.6775,60.,30.92));
#2672=CARTESIAN_POINT('Origin',(1.555,30.,29.08));
#2673=CARTESIAN_POINT('',(1.8,0.,29.08));
#2674=CARTESIAN_POINT('',(0.7775,0.,29.08));
#2675=CARTESIAN_POINT('',(1.8,15.,29.08));
#2676=CARTESIAN_POINT('Origin',(1.555,30.,29.08));
#2677=CARTESIAN_POINT('',(1.8,60.,29.08));
#2678=CARTESIAN_POINT('',(1.8,15.,29.08));
#2679=CARTESIAN_POINT('',(1.6775,60.,29.08));
#2680=CARTESIAN_POINT('Origin',(1.8,0.,0.));
#2681=CARTESIAN_POINT('',(1.8,0.,1.82));
#2682=CARTESIAN_POINT('',(1.8,0.,0.));
#2683=CARTESIAN_POINT('',(1.8,15.,1.82));
#2684=CARTESIAN_POINT('Origin',(1.8,0.,0.));
#2685=CARTESIAN_POINT('',(1.8,60.,1.82));
#2686=CARTESIAN_POINT('',(1.8,15.,1.82));
#2687=CARTESIAN_POINT('',(1.8,60.,0.));
#2688=CARTESIAN_POINT('Origin',(1.555,30.,1.82));
#2689=CARTESIAN_POINT('',(0.7775,0.,1.82));
#2690=CARTESIAN_POINT('Origin',(1.555,30.,1.82));
#2691=CARTESIAN_POINT('',(1.6775,60.,1.82));
#2692=CARTESIAN_POINT('Origin',(1.8,60.,0.));
#2693=CARTESIAN_POINT('',(0.,60.,0.));
#2694=CARTESIAN_POINT('',(1.8,60.,0.));
#2695=CARTESIAN_POINT('',(0.,60.,180.));
#2696=CARTESIAN_POINT('',(0.,60.,0.));
#2697=CARTESIAN_POINT('',(1.8,60.,180.));
#2698=CARTESIAN_POINT('Origin',(0.9,30.,0.));
#2699=CARTESIAN_POINT('',(0.,0.,0.));
#2700=CARTESIAN_POINT('',(0.,0.,0.));
#2701=CARTESIAN_POINT('',(0.,60.,0.));
#2702=CARTESIAN_POINT('Origin',(0.,0.,0.));
#2703=CARTESIAN_POINT('',(0.,0.,180.));
#2704=CARTESIAN_POINT('',(0.,0.,180.));
#2705=CARTESIAN_POINT('',(0.,0.,0.));
#2706=CARTESIAN_POINT('Origin',(0.,60.,0.));
#2707=CARTESIAN_POINT('',(0.,60.,180.));
#2708=CARTESIAN_POINT('Origin',(0.9,30.,180.));
#2848=UNCERTAINTY_MEASURE_WITH_UNIT(LENGTH_MEASURE(0.001),#2861,
'DISTANCE_ACCURACY_VALUE',
'Maximum model space distance between geometric entities at asserted c
onnectivities');
#2853=UNCERTAINTY_MEASURE_WITH_UNIT(LENGTH_MEASURE(0.001),#2861,
'DISTANCE_ACCURACY_VALUE',
'Maximum model space distance between geometric entities at asserted c
onnectivities');
#2855=(
GEOMETRIC_REPRESENTATION_CONTEXT(3)
GLOBAL_UNCERTAINTY_ASSIGNED_CONTEXT((#2848))
GLOBAL_UNIT_ASSIGNED_CONTEXT((#2861,#2863,#2864))
REPRESENTATION_CONTEXT('','3D')
);
#2860=(
GEOMETRIC_REPRESENTATION_CONTEXT(3)
GLOBAL_UNCERTAINTY_ASSIGNED_CONTEXT((#2853))
GLOBAL_UNIT_ASSIGNED_CONTEXT((#2861,#2863,#2864))
REPRESENTATION_CONTEXT('','3D')
);
#2861=(
LENGTH_UNIT()
NAMED_UNIT(*)
SI_UNIT(.CENTI.,.METRE.)
);
#2863=(
NAMED_UNIT(*)
PLANE_ANGLE_UNIT()
SI_UNIT($,.RADIAN.)
);
#2864=(
NAMED_UNIT(*)
SI_UNIT($,.STERADIAN.)
SOLID_ANGLE_UNIT()
);
#2866=SHAPE_DEFINITION_REPRESENTATION(#2872,#2902);
#2872=PRODUCT_DEFINITION_SHAPE('',$,#2909);
#2902=SHAPE_REPRESENTATION('',(#1776),#2855);
#2907=PRODUCT_DEFINITION_CONTEXT('part definition',#2927,'design');
#2909=PRODUCT_DEFINITION('Universal side panel','Universal side panel',
#2915,#2907);
#2915=PRODUCT_DEFINITION_FORMATION('',$,#2930);
#2927=APPLICATION_CONTEXT(
'Core Data for Automotive Mechanical Design Process');
#2928=PRODUCT_CONTEXT('part definition',#2927,'mechanical');
#2930=PRODUCT('Universal side panel','Universal side panel',$,(#2928));
#2936=PRESENTATION_STYLE_ASSIGNMENT((#2942));
#2942=SURFACE_STYLE_USAGE(.BOTH.,#2948);
#2948=SURFACE_SIDE_STYLE('',(#2954));
#2954=SURFACE_STYLE_FILL_AREA(#2960);
#2960=FILL_AREA_STYLE('Universal side panel finish',(#2966));
#2966=FILL_AREA_STYLE_COLOUR('Universal side panel finish',#2972);
#2972=COLOUR_RGB('Universal side panel finish',0.0941176470588235,0.231372549019608,
0.431372549019608);
ENDSEC;
END-ISO-10303-21;
